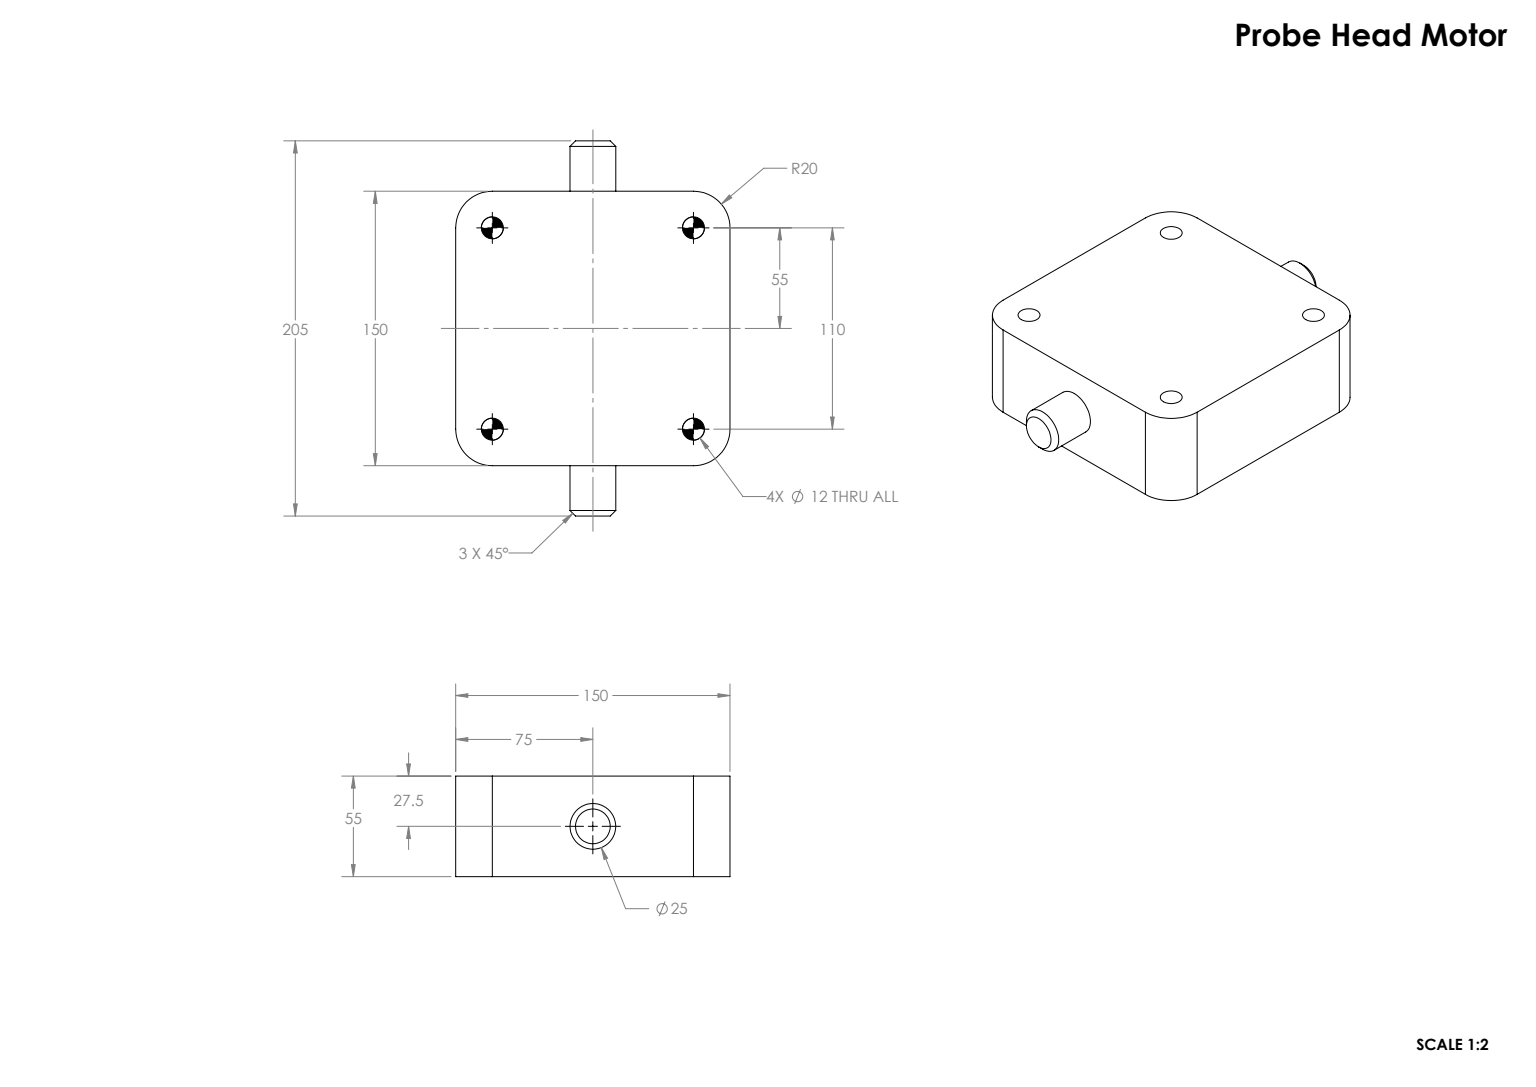
ISO-10303-21;
HEADER;
FILE_DESCRIPTION (('STEP AP214'),
    '1' );
FILE_NAME ('Probe head motor.step',
    '2026-10-28T15:55:38',
    ( '' ),
    ( '' ),
    'SwSTEP 2.0',
    'SolidWorks 2025',
    '' );
FILE_SCHEMA (( 'AUTOMOTIVE_DESIGN' ));
ENDSEC;

DATA;
#16=EDGE_LOOP ( 'NONE', ( #280, #1989 ) ) ;
#35=DIRECTION ( 'NONE',  ( 1.000000000000000000, 0.000000000000000000, 0.000000000000000000 ) ) ;
#37=DIRECTION ( 'NONE',  ( -0.000000000000000000, -0.000000000000000000, 1.000000000000000000 ) ) ;
#50=VECTOR ( 'NONE', #966, 1000.000000000000000 ) ;
#53=CARTESIAN_POINT ( 'NONE',  ( 54.99999999999999289, -55.00000000000000711, 27.50000000000000000 ) ) ;
#58=DIRECTION ( 'NONE',  ( 1.000000000000000000, 0.000000000000000000, 0.000000000000000000 ) ) ;
#59=ORIENTED_EDGE ( 'NONE', *, *, #4247, .T. ) ;
#60=CARTESIAN_POINT ( 'NONE',  ( -75.00000000000000000, 0.000000000000000000, 0.000000000000000000 ) ) ;
#66=VERTEX_POINT ( 'NONE', #5954 ) ;
#75=DIRECTION ( 'NONE',  ( -0.000000000000000000, -0.000000000000000000, -1.000000000000000000 ) ) ;
#86=CIRCLE ( 'NONE', #779, 5.999999999999984901 ) ;
#101=ORIENTED_EDGE ( 'NONE', *, *, #2517, .F. ) ;
#110=VERTEX_POINT ( 'NONE', #3400 ) ;
#138=EDGE_LOOP ( 'NONE', ( #2116, #5136, #6924, #3116 ) ) ;
#142=ORIENTED_EDGE ( 'NONE', *, *, #1025, .T. ) ;
#158=PLANE ( 'NONE',  #296 ) ;
#191=ORIENTED_EDGE ( 'NONE', *, *, #863, .F. ) ;
#192=DIRECTION ( 'NONE',  ( 1.000000000000000000, 0.000000000000000000, 0.000000000000000000 ) ) ;
#200=CARTESIAN_POINT ( 'NONE',  ( 75.00000000000000000, 55.00000000000000711, 27.50000000000000000 ) ) ;
#209=AXIS2_PLACEMENT_3D ( 'NONE', #1275, #5067, #1401 ) ;
#220=DIRECTION ( 'NONE',  ( 1.000000000000000000, 0.000000000000000000, 0.000000000000000000 ) ) ;
#236=CIRCLE ( 'NONE', #5782, 12.50000000000000000 ) ;
#241=EDGE_CURVE ( 'NONE', #7110, #7555, #6784, .T. ) ;
#246=FACE_OUTER_BOUND ( 'NONE', #495, .T. ) ;
#257=LINE ( 'NONE', #1580, #7553 ) ;
#275=ORIENTED_EDGE ( 'NONE', *, *, #5871, .F. ) ;
#277=AXIS2_PLACEMENT_3D ( 'NONE', #5185, #677, #1430 ) ;
#280=ORIENTED_EDGE ( 'NONE', *, *, #241, .T. ) ;
#288=DIRECTION ( 'NONE',  ( 0.000000000000000000, 0.000000000000000000, 1.000000000000000000 ) ) ;
#296=AXIS2_PLACEMENT_3D ( 'NONE', #5951, #1969, #3246 ) ;
#301=ORIENTED_EDGE ( 'NONE', *, *, #715, .F. ) ;
#316=CARTESIAN_POINT ( 'NONE',  ( 54.99999999999999289, 55.00000000000000711, 27.50000000000000000 ) ) ;
#339=CARTESIAN_POINT ( 'NONE',  ( -75.00000000000000000, -75.00000000000000000, -27.50000000000000000 ) ) ;
#340=ORIENTED_EDGE ( 'NONE', *, *, #1134, .T. ) ;
#356=AXIS2_PLACEMENT_3D ( 'NONE', #3494, #2749, #5417 ) ;
#382=CARTESIAN_POINT ( 'NONE',  ( -54.99999999999999289, 55.00000000000000711, 27.50000000000000000 ) ) ;
#384=CIRCLE ( 'NONE', #1751, 5.999999999999984901 ) ;
#388=ORIENTED_EDGE ( 'NONE', *, *, #3277, .T. ) ;
#395=DIRECTION ( 'NONE',  ( -0.000000000000000000, -0.000000000000000000, 1.000000000000000000 ) ) ;
#420=CARTESIAN_POINT ( 'NONE',  ( -102.5000000000000000, 0.000000000000000000, -9.500000000000008882 ) ) ;
#437=DIRECTION ( 'NONE',  ( 0.000000000000000000, 0.000000000000000000, -1.000000000000000000 ) ) ;
#453=CARTESIAN_POINT ( 'NONE',  ( -75.00000000000000000, 55.00000000000000711, 27.50000000000000000 ) ) ;
#494=CARTESIAN_POINT ( 'NONE',  ( -75.00000000000000000, 1.530808498934191521E-15, -12.50000000000000000 ) ) ;
#495=EDGE_LOOP ( 'NONE', ( #2773, #191, #1926, #6706 ) ) ;
#499=ORIENTED_EDGE ( 'NONE', *, *, #1382, .F. ) ;
#512=EDGE_CURVE ( 'NONE', #554, #2252, #3311, .T. ) ;
#518=FACE_OUTER_BOUND ( 'NONE', #6089, .T. ) ;
#527=CARTESIAN_POINT ( 'NONE',  ( 54.99999999999999289, -55.00000000000000711, -27.50000000000000000 ) ) ;
#531=DIRECTION ( 'NONE',  ( 1.000000000000000000, 0.000000000000000000, 0.000000000000000000 ) ) ;
#532=DIRECTION ( 'NONE',  ( 0.000000000000000000, 0.000000000000000000, -1.000000000000000000 ) ) ;
#550=SHAPE_DEFINITION_REPRESENTATION ( #6549, #5477 ) ;
#554=VERTEX_POINT ( 'NONE', #494 ) ;
#582=DIRECTION ( 'NONE',  ( 0.7071067811865487940, 0.000000000000000000, -0.7071067811865463515 ) ) ;
#585=ORIENTED_EDGE ( 'NONE', *, *, #8135, .F. ) ;
#596=ORIENTED_EDGE ( 'NONE', *, *, #2034, .T. ) ;
#598=AXIS2_PLACEMENT_3D ( 'NONE', #1970, #37, #7220 ) ;
#614=DIRECTION ( 'NONE',  ( 1.000000000000000000, 0.000000000000000000, 0.000000000000000000 ) ) ;
#617=ADVANCED_FACE ( 'NONE', ( #5555 ), #6947, .T. ) ;
#641=ORIENTED_EDGE ( 'NONE', *, *, #6036, .F. ) ;
#652=AXIS2_PLACEMENT_3D ( 'NONE', #316, #3056, #8044 ) ;
#674=FACE_OUTER_BOUND ( 'NONE', #5673, .T. ) ;
#677=DIRECTION ( 'NONE',  ( 1.000000000000000000, 0.000000000000000000, 0.000000000000000000 ) ) ;
#693=FACE_OUTER_BOUND ( 'NONE', #2495, .T. ) ;
#715=EDGE_CURVE ( 'NONE', #3072, #2500, #2204, .T. ) ;
#723=ORIENTED_EDGE ( 'NONE', *, *, #8302, .T. ) ;
#734=EDGE_LOOP ( 'NONE', ( #5853, #4869 ) ) ;
#752=CARTESIAN_POINT ( 'NONE',  ( -54.99999999999999289, 75.00000000000000000, 27.50000000000000000 ) ) ;
#760=ORIENTED_EDGE ( 'NONE', *, *, #7716, .F. ) ;
#764=EDGE_LOOP ( 'NONE', ( #7104, #4270, #4312, #1914 ) ) ;
#773=CYLINDRICAL_SURFACE ( 'NONE', #4839, 5.999999999999991118 ) ;
#779=AXIS2_PLACEMENT_3D ( 'NONE', #7723, #2681, #5258 ) ;
#796=ORIENTED_EDGE ( 'NONE', *, *, #4247, .F. ) ;
#807=CONICAL_SURFACE ( 'NONE', #951, 12.50000000000000000, 0.7853981633974560506 ) ;
#808=AXIS2_PLACEMENT_3D ( 'NONE', #888, #4718, #2129 ) ;
#812=ORIENTED_EDGE ( 'NONE', *, *, #1185, .F. ) ;
#828=CARTESIAN_POINT ( 'NONE',  ( 75.00000000000000000, 55.00000000000000711, -27.50000000000000000 ) ) ;
#836=VERTEX_POINT ( 'NONE', #6820 ) ;
#847=DIRECTION ( 'NONE',  ( 0.000000000000000000, 0.000000000000000000, 1.000000000000000000 ) ) ;
#848=CIRCLE ( 'NONE', #1394, 5.999999999999991118 ) ;
#863=EDGE_CURVE ( 'NONE', #7276, #4717, #4483, .T. ) ;
#885=EDGE_CURVE ( 'NONE', #1626, #6639, #3839, .T. ) ;
#888=CARTESIAN_POINT ( 'NONE',  ( -54.99999999999999289, -55.00000000000000711, 27.50000000000000000 ) ) ;
#912=CARTESIAN_POINT ( 'NONE',  ( -54.99999999999999289, 55.00000000000000711, -27.50000000000000000 ) ) ;
#914=ORIENTED_EDGE ( 'NONE', *, *, #3174, .T. ) ;
#921=EDGE_CURVE ( 'NONE', #3696, #7524, #4657, .T. ) ;
#928=CIRCLE ( 'NONE', #1205, 5.999999999999991118 ) ;
#951=AXIS2_PLACEMENT_3D ( 'NONE', #3629, #2188, #7493 ) ;
#956=EDGE_LOOP ( 'NONE', ( #1669, #2525 ) ) ;
#965=DIRECTION ( 'NONE',  ( -1.000000000000000000, 0.000000000000000000, 0.000000000000000000 ) ) ;
#966=DIRECTION ( 'NONE',  ( -0.000000000000000000, -0.000000000000000000, 1.000000000000000000 ) ) ;
#976=ORIENTED_EDGE ( 'NONE', *, *, #1235, .T. ) ;
#988=DIRECTION ( 'NONE',  ( -0.000000000000000000, -0.000000000000000000, 1.000000000000000000 ) ) ;
#1025=EDGE_CURVE ( 'NONE', #6358, #4954, #6815, .T. ) ;
#1060=AXIS2_PLACEMENT_3D ( 'NONE', #3558, #6825, #1679 ) ;
#1064=ORIENTED_EDGE ( 'NONE', *, *, #1543, .F. ) ;
#1066=AXIS2_PLACEMENT_3D ( 'NONE', #60, #2652, #5223 ) ;
#1068=CARTESIAN_POINT ( 'NONE',  ( -60.99999999999998579, -55.00000000000000711, 27.50000000000000000 ) ) ;
#1073=AXIS2_PLACEMENT_3D ( 'NONE', #4907, #6004, #220 ) ;
#1075=ADVANCED_FACE ( 'NONE', ( #7748 ), #1882, .T. ) ;
#1117=LINE ( 'NONE', #2431, #6840 ) ;
#1134=EDGE_CURVE ( 'NONE', #5699, #3094, #5750, .T. ) ;
#1149=DIRECTION ( 'NONE',  ( -1.000000000000000000, 0.000000000000000000, 0.000000000000000000 ) ) ;
#1152=CARTESIAN_POINT ( 'NONE',  ( 60.99999999999998579, -55.00000000000000711, 27.50000000000000000 ) ) ;
#1159=PLANE ( 'NONE',  #4129 ) ;
#1169=CARTESIAN_POINT ( 'NONE',  ( 102.5000000000000000, 0.000000000000000000, 12.50000000000000000 ) ) ;
#1177=CIRCLE ( 'NONE', #2781, 5.999999999999984901 ) ;
#1185=EDGE_CURVE ( 'NONE', #8175, #4245, #7456, .T. ) ;
#1205=AXIS2_PLACEMENT_3D ( 'NONE', #2733, #7214, #192 ) ;
#1214=AXIS2_PLACEMENT_3D ( 'NONE', #912, #6734, #4258 ) ;
#1216=DIRECTION ( 'NONE',  ( -1.000000000000000000, 0.000000000000000000, 0.000000000000000000 ) ) ;
#1222=VECTOR ( 'NONE', #4044, 1000.000000000000000 ) ;
#1235=EDGE_CURVE ( 'NONE', #6452, #7276, #5560, .T. ) ;
#1275=CARTESIAN_POINT ( 'NONE',  ( -102.5000000000000000, 0.000000000000000000, 0.000000000000000000 ) ) ;
#1292=DIRECTION ( 'NONE',  ( -0.000000000000000000, -0.000000000000000000, 1.000000000000000000 ) ) ;
#1295=EDGE_LOOP ( 'NONE', ( #5051, #4898, #3815, #4605 ) ) ;
#1299=AXIS2_PLACEMENT_3D ( 'NONE', #5884, #1507, #5927 ) ;
#1309=STYLED_ITEM('',(#8386),#3442);
#1316=ORIENTED_EDGE ( 'NONE', *, *, #5149, .T. ) ;
#1341=EDGE_LOOP ( 'NONE', ( #3743, #2060, #2905, #3577 ) ) ;
#1361=CARTESIAN_POINT ( 'NONE',  ( -102.5000000000000000, 1.347111479062088996E-15, 9.500000000000008882 ) ) ;
#1363=ORIENTED_EDGE ( 'NONE', *, *, #7635, .T. ) ;
#1377=DIRECTION ( 'NONE',  ( 0.000000000000000000, 0.000000000000000000, -1.000000000000000000 ) ) ;
#1378=CYLINDRICAL_SURFACE ( 'NONE', #2162, 5.999999999999991118 ) ;
#1382=EDGE_CURVE ( 'NONE', #7568, #7256, #5423, .T. ) ;
#1386=EDGE_LOOP ( 'NONE', ( #5814, #142 ) ) ;
#1392=EDGE_CURVE ( 'NONE', #4954, #2252, #6357, .T. ) ;
#1394=AXIS2_PLACEMENT_3D ( 'NONE', #2395, #3731, #6308 ) ;
#1398=ORIENTED_EDGE ( 'NONE', *, *, #1382, .T. ) ;
#1399=DIRECTION ( 'NONE',  ( -0.000000000000000000, -0.000000000000000000, 1.000000000000000000 ) ) ;
#1401=DIRECTION ( 'NONE',  ( 0.000000000000000000, 0.000000000000000000, 1.000000000000000000 ) ) ;
#1405=DIRECTION ( 'NONE',  ( 0.7071067811865487940, 8.659560562354918067E-17, 0.7071067811865463515 ) ) ;
#1406=FACE_OUTER_BOUND ( 'NONE', #6060, .T. ) ;
#1407=CARTESIAN_POINT ( 'NONE',  ( -75.00000000000000000, 55.00000000000000711, -27.50000000000000000 ) ) ;
#1430=DIRECTION ( 'NONE',  ( 0.000000000000000000, 0.000000000000000000, 1.000000000000000000 ) ) ;
#1433=VECTOR ( 'NONE', #5737, 1000.000000000000000 ) ;
#1434=FACE_OUTER_BOUND ( 'NONE', #2226, .T. ) ;
#1449=DIRECTION ( 'NONE',  ( 1.000000000000000000, 0.000000000000000000, -0.000000000000000000 ) ) ;
#1460=AXIS2_PLACEMENT_3D ( 'NONE', #7776, #8199, #6245 ) ;
#1461=DIRECTION ( 'NONE',  ( 1.000000000000000000, 0.000000000000000000, 0.000000000000000000 ) ) ;
#1472=VECTOR ( 'NONE', #4316, 1000.000000000000000 ) ;
#1476=EDGE_LOOP ( 'NONE', ( #4624, #1316 ) ) ;
#1482=PLANE ( 'NONE',  #4550 ) ;
#1492=DIRECTION ( 'NONE',  ( 1.000000000000000000, 0.000000000000000000, 0.000000000000000000 ) ) ;
#1498=ADVANCED_FACE ( 'NONE', ( #4662 ), #3983, .F. ) ;
#1507=DIRECTION ( 'NONE',  ( 0.000000000000000000, 0.000000000000000000, 1.000000000000000000 ) ) ;
#1523=LINE ( 'NONE', #4077, #6033 ) ;
#1542=EDGE_CURVE ( 'NONE', #7555, #4076, #4780, .T. ) ;
#1543=EDGE_CURVE ( 'NONE', #3044, #6339, #848, .T. ) ;
#1565=CARTESIAN_POINT ( 'NONE',  ( 102.5000000000000000, 0.000000000000000000, 12.50000000000000000 ) ) ;
#1572=AXIS2_PLACEMENT_3D ( 'NONE', #3282, #1924, #5869 ) ;
#1580=CARTESIAN_POINT ( 'NONE',  ( 99.49999999999998579, 1.530808498934191521E-15, -12.50000000000000000 ) ) ;
#1585=PRODUCT_DEFINITION ( 'UNKNOWN', '', #8277, #4878 ) ;
#1586=AXIS2_PLACEMENT_3D ( 'NONE', #2848, #5393, #6777 ) ;
#1589=DIRECTION ( 'NONE',  ( 1.000000000000000000, 0.000000000000000000, 0.000000000000000000 ) ) ;
#1599=AXIS2_PLACEMENT_3D ( 'NONE', #7278, #2142, #6512 ) ;
#1609=ORIENTED_EDGE ( 'NONE', *, *, #6476, .F. ) ;
#1619=ORIENTED_EDGE ( 'NONE', *, *, #2976, .F. ) ;
#1625=DIRECTION ( 'NONE',  ( 1.000000000000000000, 0.000000000000000000, 0.000000000000000000 ) ) ;
#1626=VERTEX_POINT ( 'NONE', #5552 ) ;
#1635=DIRECTION ( 'NONE',  ( -0.000000000000000000, -0.000000000000000000, -1.000000000000000000 ) ) ;
#1654=ORIENTED_EDGE ( 'NONE', *, *, #2229, .F. ) ;
#1657=ORIENTED_EDGE ( 'NONE', *, *, #1392, .T. ) ;
#1661=LINE ( 'NONE', #339, #5798 ) ;
#1663=ADVANCED_FACE ( 'NONE', ( #3888, #2011, #6544, #5286, #3359 ), #158, .F. ) ;
#1669=ORIENTED_EDGE ( 'NONE', *, *, #6182, .F. ) ;
#1675=CARTESIAN_POINT ( 'NONE',  ( -75.00000000000000000, -54.99999999999999289, 27.50000000000000000 ) ) ;
#1679=DIRECTION ( 'NONE',  ( 0.000000000000000000, 0.000000000000000000, -1.000000000000000000 ) ) ;
#1685=DIRECTION ( 'NONE',  ( -0.000000000000000000, -1.000000000000000000, -0.000000000000000000 ) ) ;
#1689=ORIENTED_EDGE ( 'NONE', *, *, #6534, .T. ) ;
#1694=DIRECTION ( 'NONE',  ( 1.000000000000000000, 0.000000000000000000, 0.000000000000000000 ) ) ;
#1696=ORIENTED_EDGE ( 'NONE', *, *, #715, .T. ) ;
#1715=CIRCLE ( 'NONE', #7657, 5.999999999999991118 ) ;
#1724=ORIENTED_EDGE ( 'NONE', *, *, #5346, .T. ) ;
#1731=EDGE_LOOP ( 'NONE', ( #7387, #5133, #8189, #1619 ) ) ;
#1749=DIRECTION ( 'NONE',  ( 1.000000000000000000, 0.000000000000000000, 0.000000000000000000 ) ) ;
#1751=AXIS2_PLACEMENT_3D ( 'NONE', #1805, #2063, #7837 ) ;
#1765=LINE ( 'NONE', #6220, #6456 ) ;
#1774=CARTESIAN_POINT ( 'NONE',  ( 102.5000000000000000, 0.000000000000000000, 12.50000000000000000 ) ) ;
#1777=FACE_OUTER_BOUND ( 'NONE', #3624, .T. ) ;
#1800=VECTOR ( 'NONE', #4904, 1000.000000000000000 ) ;
#1805=CARTESIAN_POINT ( 'NONE',  ( 54.99999999999999289, 55.00000000000000711, -27.50000000000000000 ) ) ;
#1829=ADVANCED_FACE ( 'NONE', ( #5289, #5255 ), #3937, .F. ) ;
#1867=EDGE_CURVE ( 'NONE', #8175, #3044, #4291, .T. ) ;
#1882=PLANE ( 'NONE',  #1572 ) ;
#1913=VECTOR ( 'NONE', #8057, 1000.000000000000000 ) ;
#1914=ORIENTED_EDGE ( 'NONE', *, *, #5462, .F. ) ;
#1924=DIRECTION ( 'NONE',  ( -1.000000000000000000, 0.000000000000000000, -0.000000000000000000 ) ) ;
#1926=ORIENTED_EDGE ( 'NONE', *, *, #1235, .F. ) ;
#1927=VECTOR ( 'NONE', #2123, 1000.000000000000000 ) ;
#1930=ADVANCED_FACE ( 'NONE', ( #7832 ), #6986, .T. ) ;
#1948=ORIENTED_EDGE ( 'NONE', *, *, #885, .F. ) ;
#1959=ORIENTED_EDGE ( 'NONE', *, *, #2080, .T. ) ;
#1969=DIRECTION ( 'NONE',  ( 0.000000000000000000, 0.000000000000000000, 1.000000000000000000 ) ) ;
#1970=CARTESIAN_POINT ( 'NONE',  ( 54.99999999999999289, -55.00000000000000711, -27.50000000000000000 ) ) ;
#1973=CARTESIAN_POINT ( 'NONE',  ( -49.00000000000000000, 55.00000000000000711, 27.50000000000000000 ) ) ;
#1976=EDGE_CURVE ( 'NONE', #66, #5533, #7130, .T. ) ;
#1980=EDGE_CURVE ( 'NONE', #7524, #2265, #2627, .T. ) ;
#1983=DIRECTION ( 'NONE',  ( 0.000000000000000000, 0.000000000000000000, 1.000000000000000000 ) ) ;
#1985=CARTESIAN_POINT ( 'NONE',  ( -54.99999999999999289, 55.00000000000000711, -27.50000000000000000 ) ) ;
#1989=ORIENTED_EDGE ( 'NONE', *, *, #4023, .T. ) ;
#1996=CIRCLE ( 'NONE', #3715, 12.50000000000000000 ) ;
#2000=CARTESIAN_POINT ( 'NONE',  ( -54.99999999999999289, 55.00000000000000711, -27.50000000000000000 ) ) ;
#2011=FACE_BOUND ( 'NONE', #2386, .T. ) ;
#2018=ADVANCED_FACE ( 'NONE', ( #4678, #7262 ), #1482, .F. ) ;
#2028=AXIS2_PLACEMENT_3D ( 'NONE', #8099, #3603, #7469 ) ;
#2034=EDGE_CURVE ( 'NONE', #6639, #2500, #5444, .T. ) ;
#2047=CARTESIAN_POINT ( 'NONE',  ( -60.99999999999998579, -55.00000000000000711, 27.50000000000000000 ) ) ;
#2053=DIRECTION ( 'NONE',  ( -1.000000000000000000, -0.000000000000000000, -0.000000000000000000 ) ) ;
#2060=ORIENTED_EDGE ( 'NONE', *, *, #6540, .T. ) ;
#2063=DIRECTION ( 'NONE',  ( -0.000000000000000000, -0.000000000000000000, 1.000000000000000000 ) ) ;
#2066=ORIENTED_EDGE ( 'NONE', *, *, #7515, .F. ) ;
#2076=CARTESIAN_POINT ( 'NONE',  ( 75.00000000000000000, 0.000000000000000000, 0.000000000000000000 ) ) ;
#2080=EDGE_CURVE ( 'NONE', #3696, #2372, #2373, .T. ) ;
#2110=CARTESIAN_POINT ( 'NONE',  ( -60.99999999999997868, 55.00000000000000711, -27.50000000000000000 ) ) ;
#2116=ORIENTED_EDGE ( 'NONE', *, *, #4902, .F. ) ;
#2123=DIRECTION ( 'NONE',  ( 0.000000000000000000, 1.000000000000000000, 0.000000000000000000 ) ) ;
#2126=DIRECTION ( 'NONE',  ( -1.000000000000000000, -0.000000000000000000, -0.000000000000000000 ) ) ;
#2129=DIRECTION ( 'NONE',  ( 1.000000000000000000, 0.000000000000000000, 0.000000000000000000 ) ) ;
#2134=AXIS2_PLACEMENT_3D ( 'NONE', #8300, #6470, #614 ) ;
#2138=DIRECTION ( 'NONE',  ( 1.000000000000000000, 0.000000000000000000, 0.000000000000000000 ) ) ;
#2142=DIRECTION ( 'NONE',  ( 1.000000000000000000, 0.000000000000000000, 0.000000000000000000 ) ) ;
#2146=( NAMED_UNIT ( * ) SI_UNIT ( $, .STERADIAN. ) SOLID_ANGLE_UNIT ( ) );
#2150=ORIENTED_EDGE ( 'NONE', *, *, #1542, .F. ) ;
#2162=AXIS2_PLACEMENT_3D ( 'NONE', #53, #5882, #7285 ) ;
#2166=DIRECTION ( 'NONE',  ( 0.000000000000000000, 0.000000000000000000, 1.000000000000000000 ) ) ;
#2188=DIRECTION ( 'NONE',  ( -1.000000000000000000, -0.000000000000000000, -0.000000000000000000 ) ) ;
#2195=DIRECTION ( 'NONE',  ( -0.000000000000000000, -0.000000000000000000, 1.000000000000000000 ) ) ;
#2202=DIRECTION ( 'NONE',  ( -0.000000000000000000, -1.000000000000000000, -0.000000000000000000 ) ) ;
#2204=LINE ( 'NONE', #1675, #50 ) ;
#2223=FACE_BOUND ( 'NONE', #7249, .T. ) ;
#2226=EDGE_LOOP ( 'NONE', ( #2246, #7149, #4337, #6802 ) ) ;
#2229=EDGE_CURVE ( 'NONE', #5699, #7276, #6330, .T. ) ;
#2235=ORIENTED_EDGE ( 'NONE', *, *, #1867, .T. ) ;
#2246=ORIENTED_EDGE ( 'NONE', *, *, #6540, .F. ) ;
#2252=VERTEX_POINT ( 'NONE', #4669 ) ;
#2265=VERTEX_POINT ( 'NONE', #7253 ) ;
#2267=DIRECTION ( 'NONE',  ( 0.000000000000000000, 1.000000000000000000, 0.000000000000000000 ) ) ;
#2269=CARTESIAN_POINT ( 'NONE',  ( -54.99999999999999289, -54.99999999999999289, 27.50000000000000000 ) ) ;
#2270=EDGE_LOOP ( 'NONE', ( #5470, #1064 ) ) ;
#2315=CYLINDRICAL_SURFACE ( 'NONE', #1073, 5.999999999999991118 ) ;
#2337=AXIS2_PLACEMENT_3D ( 'NONE', #3997, #5908, #4801 ) ;
#2345=EDGE_CURVE ( 'NONE', #2252, #7231, #4050, .T. ) ;
#2346=EDGE_LOOP ( 'NONE', ( #8111, #6761 ) ) ;
#2348=EDGE_CURVE ( 'NONE', #6145, #8000, #1996, .T. ) ;
#2372=VERTEX_POINT ( 'NONE', #5312 ) ;
#2373=LINE ( 'NONE', #3563, #1913 ) ;
#2384=ORIENTED_EDGE ( 'NONE', *, *, #4773, .F. ) ;
#2386=EDGE_LOOP ( 'NONE', ( #59, #3390 ) ) ;
#2395=CARTESIAN_POINT ( 'NONE',  ( -54.99999999999999289, -55.00000000000000711, 27.50000000000000000 ) ) ;
#2431=CARTESIAN_POINT ( 'NONE',  ( -75.00000000000000000, 75.00000000000000000, 27.50000000000000000 ) ) ;
#2435=ORIENTED_EDGE ( 'NONE', *, *, #8135, .T. ) ;
#2456=DIRECTION ( 'NONE',  ( -0.7071067811865420216, 0.000000000000000000, 0.7071067811865531239 ) ) ;
#2463=ORIENTED_EDGE ( 'NONE', *, *, #1980, .T. ) ;
#2465=ORIENTED_EDGE ( 'NONE', *, *, #3174, .F. ) ;
#2466=CARTESIAN_POINT ( 'NONE',  ( -49.00000000000000000, -55.00000000000000711, 27.50000000000000000 ) ) ;
#2480=CARTESIAN_POINT ( 'NONE',  ( -75.00000000000000000, 0.000000000000000000, 12.50000000000000000 ) ) ;
#2488=DIRECTION ( 'NONE',  ( -0.000000000000000000, -0.000000000000000000, 1.000000000000000000 ) ) ;
#2495=EDGE_LOOP ( 'NONE', ( #4227, #7457, #7004, #2728 ) ) ;
#2500=VERTEX_POINT ( 'NONE', #7466 ) ;
#2517=EDGE_CURVE ( 'NONE', #4954, #6358, #2712, .T. ) ;
#2525=ORIENTED_EDGE ( 'NONE', *, *, #3782, .F. ) ;
#2526=CARTESIAN_POINT ( 'NONE',  ( -102.5000000000000000, 0.000000000000000000, -9.500000000000008882 ) ) ;
#2538=CIRCLE ( 'NONE', #7244, 5.999999999999991118 ) ;
#2558=ORIENTED_EDGE ( 'NONE', *, *, #3873, .F. ) ;
#2595=LINE ( 'NONE', #1973, #6878 ) ;
#2627=LINE ( 'NONE', #3996, #2932 ) ;
#2635=DIRECTION ( 'NONE',  ( -0.000000000000000000, -0.000000000000000000, 1.000000000000000000 ) ) ;
#2652=DIRECTION ( 'NONE',  ( 1.000000000000000000, 0.000000000000000000, 0.000000000000000000 ) ) ;
#2656=CARTESIAN_POINT ( 'NONE',  ( 55.00000000000000711, -75.00000000000000000, -27.50000000000000000 ) ) ;
#2664=DIRECTION ( 'NONE',  ( 0.000000000000000000, 0.000000000000000000, 1.000000000000000000 ) ) ;
#2673=CARTESIAN_POINT ( 'NONE',  ( 102.5000000000000000, 0.000000000000000000, 0.000000000000000000 ) ) ;
#2677=AXIS2_PLACEMENT_3D ( 'NONE', #4426, #7098, #5199 ) ;
#2681=DIRECTION ( 'NONE',  ( -0.000000000000000000, -0.000000000000000000, 1.000000000000000000 ) ) ;
#2686=AXIS2_PLACEMENT_3D ( 'NONE', #3148, #3792, #6322 ) ;
#2699=CIRCLE ( 'NONE', #808, 5.999999999999991118 ) ;
#2712=CIRCLE ( 'NONE', #1586, 9.500000000000008882 ) ;
#2722=CARTESIAN_POINT ( 'NONE',  ( 49.00000000000000000, -55.00000000000000711, 27.50000000000000000 ) ) ;
#2728=ORIENTED_EDGE ( 'NONE', *, *, #3761, .F. ) ;
#2731=LINE ( 'NONE', #752, #7531 ) ;
#2733=CARTESIAN_POINT ( 'NONE',  ( 54.99999999999999289, -55.00000000000000711, 27.50000000000000000 ) ) ;
#2737=CARTESIAN_POINT ( 'NONE',  ( 54.99999999999999289, -54.99999999999999289, 27.50000000000000000 ) ) ;
#2749=DIRECTION ( 'NONE',  ( 0.000000000000000000, 0.000000000000000000, 1.000000000000000000 ) ) ;
#2773=ORIENTED_EDGE ( 'NONE', *, *, #4299, .F. ) ;
#2781=AXIS2_PLACEMENT_3D ( 'NONE', #527, #395, #4256 ) ;
#2799=CONICAL_SURFACE ( 'NONE', #8058, 12.50000000000000000, 0.7853981633974560506 ) ;
#2801=AXIS2_PLACEMENT_3D ( 'NONE', #5240, #3928, #6497 ) ;
#2808=VECTOR ( 'NONE', #2456, 999.9999999999998863 ) ;
#2817=LINE ( 'NONE', #1565, #4522 ) ;
#2818=CIRCLE ( 'NONE', #7413, 5.999999999999991118 ) ;
#2819=AXIS2_PLACEMENT_3D ( 'NONE', #6539, #3393, #3314 ) ;
#2824=AXIS2_PLACEMENT_3D ( 'NONE', #2000, #8279, #4534 ) ;
#2827=DIRECTION ( 'NONE',  ( -0.000000000000000000, -0.000000000000000000, 1.000000000000000000 ) ) ;
#2829=CARTESIAN_POINT ( 'NONE',  ( -60.99999999999998579, 55.00000000000000711, 27.50000000000000000 ) ) ;
#2848=CARTESIAN_POINT ( 'NONE',  ( -102.5000000000000000, 0.000000000000000000, 0.000000000000000000 ) ) ;
#2856=EDGE_LOOP ( 'NONE', ( #7495, #6405, #5755, #3429 ) ) ;
#2863=DIRECTION ( 'NONE',  ( 1.000000000000000000, 0.000000000000000000, 0.000000000000000000 ) ) ;
#2878=AXIS2_PLACEMENT_3D ( 'NONE', #6082, #4777, #6611 ) ;
#2883=CARTESIAN_POINT ( 'NONE',  ( -54.99999999999999289, -54.99999999999999289, -27.50000000000000000 ) ) ;
#2894=CARTESIAN_POINT ( 'NONE',  ( 54.99999999999999289, 55.00000000000000711, 27.50000000000000000 ) ) ;
#2905=ORIENTED_EDGE ( 'NONE', *, *, #2348, .F. ) ;
#2911=DIRECTION ( 'NONE',  ( 1.000000000000000000, 0.000000000000000000, 0.000000000000000000 ) ) ;
#2932=VECTOR ( 'NONE', #1399, 1000.000000000000000 ) ;
#2941=ORIENTED_EDGE ( 'NONE', *, *, #5514, .F. ) ;
#2976=EDGE_CURVE ( 'NONE', #7110, #8191, #5228, .T. ) ;
#2985=ORIENTED_EDGE ( 'NONE', *, *, #241, .F. ) ;
#2992=CARTESIAN_POINT ( 'NONE',  ( 55.00000000000000711, 75.00000000000000000, 27.50000000000000000 ) ) ;
#3044=VERTEX_POINT ( 'NONE', #2047 ) ;
#3055=CYLINDRICAL_SURFACE ( 'NONE', #6596, 20.00000000000000355 ) ;
#3056=DIRECTION ( 'NONE',  ( -0.000000000000000000, -0.000000000000000000, 1.000000000000000000 ) ) ;
#3072=VERTEX_POINT ( 'NONE', #3670 ) ;
#3074=ADVANCED_FACE ( 'NONE', ( #674 ), #7169, .F. ) ;
#3088=ORIENTED_EDGE ( 'NONE', *, *, #1025, .F. ) ;
#3094=VERTEX_POINT ( 'NONE', #2656 ) ;
#3100=ORIENTED_EDGE ( 'NONE', *, *, #6902, .F. ) ;
#3101=VECTOR ( 'NONE', #1685, 1000.000000000000000 ) ;
#3105=DIRECTION ( 'NONE',  ( 0.000000000000000000, 0.000000000000000000, -1.000000000000000000 ) ) ;
#3116=ORIENTED_EDGE ( 'NONE', *, *, #4151, .T. ) ;
#3139=CARTESIAN_POINT ( 'NONE',  ( 102.5000000000000000, 1.347111479062085446E-15, -9.499999999999952038 ) ) ;
#3148=CARTESIAN_POINT ( 'NONE',  ( -99.49999999999998579, 0.000000000000000000, 0.000000000000000000 ) ) ;
#3151=LINE ( 'NONE', #3748, #1433 ) ;
#3171=CIRCLE ( 'NONE', #7910, 5.999999999999984901 ) ;
#3173=CONICAL_SURFACE ( 'NONE', #7653, 9.500000000000008882, 0.7853981633974466137 ) ;
#3174=EDGE_CURVE ( 'NONE', #7809, #1626, #2731, .T. ) ;
#3186=EDGE_LOOP ( 'NONE', ( #3088, #6469, #3532, #4873 ) ) ;
#3221=VECTOR ( 'NONE', #5579, 1000.000000000000000 ) ;
#3246=DIRECTION ( 'NONE',  ( 1.000000000000000000, 0.000000000000000000, -0.000000000000000000 ) ) ;
#3249=CYLINDRICAL_SURFACE ( 'NONE', #3777, 12.50000000000000000 ) ;
#3262=ORIENTED_EDGE ( 'NONE', *, *, #4902, .T. ) ;
#3277=EDGE_CURVE ( 'NONE', #7206, #3072, #6028, .T. ) ;
#3280=CARTESIAN_POINT ( 'NONE',  ( -49.00000000000000711, 55.00000000000000711, -27.50000000000000000 ) ) ;
#3282=CARTESIAN_POINT ( 'NONE',  ( -102.5000000000000000, 0.000000000000000000, 12.50000000000000000 ) ) ;
#3286=ADVANCED_FACE ( 'NONE', ( #5558 ), #7591, .F. ) ;
#3295=ADVANCED_FACE ( 'NONE', ( #3553 ), #4311, .T. ) ;
#3311=LINE ( 'NONE', #3700, #3405 ) ;
#3314=DIRECTION ( 'NONE',  ( 0.000000000000000000, 0.000000000000000000, -1.000000000000000000 ) ) ;
#3322=CARTESIAN_POINT ( 'NONE',  ( -102.5000000000000000, 1.163414459189986668E-15, 9.500000000000008882 ) ) ;
#3324=AXIS2_PLACEMENT_3D ( 'NONE', #7462, #5642, #965 ) ;
#3325=CARTESIAN_POINT ( 'NONE',  ( 0.000000000000000000, 0.000000000000000000, 27.50000000000000000 ) ) ;
#3348=CIRCLE ( 'NONE', #3904, 20.00000000000000355 ) ;
#3359=FACE_OUTER_BOUND ( 'NONE', #5904, .T. ) ;
#3368=ORIENTED_EDGE ( 'NONE', *, *, #7209, .F. ) ;
#3371=FACE_OUTER_BOUND ( 'NONE', #2856, .T. ) ;
#3378=ADVANCED_FACE ( 'NONE', ( #3822 ), #3173, .T. ) ;
#3379=( NAMED_UNIT ( * ) SI_UNIT ( $, .STERADIAN. ) SOLID_ANGLE_UNIT ( ) );
#3390=ORIENTED_EDGE ( 'NONE', *, *, #1185, .T. ) ;
#3393=DIRECTION ( 'NONE',  ( -1.000000000000000000, -0.000000000000000000, -0.000000000000000000 ) ) ;
#3400=CARTESIAN_POINT ( 'NONE',  ( 55.00000000000000711, 75.00000000000000000, 27.50000000000000000 ) ) ;
#3405=VECTOR ( 'NONE', #4363, 1000.000000000000000 ) ;
#3424=CARTESIAN_POINT ( 'NONE',  ( -75.00000000000000000, -75.00000000000000000, -27.50000000000000000 ) ) ;
#3429=ORIENTED_EDGE ( 'NONE', *, *, #3873, .T. ) ;
#3436=DIRECTION ( 'NONE',  ( 1.000000000000000000, 0.000000000000000000, 0.000000000000000000 ) ) ;
#3442=MANIFOLD_SOLID_BREP ( 'Chamfer1', #5981 ) ;
#3446=CARTESIAN_POINT ( 'NONE',  ( -54.99999999999999289, -75.00000000000000000, 27.50000000000000000 ) ) ;
#3453=CARTESIAN_POINT ( 'NONE',  ( 49.00000000000000711, 55.00000000000000711, -27.50000000000000000 ) ) ;
#3494=CARTESIAN_POINT ( 'NONE',  ( 55.00000000000000711, 54.99999999999999289, 27.50000000000000000 ) ) ;
#3532=ORIENTED_EDGE ( 'NONE', *, *, #2345, .F. ) ;
#3541=DIRECTION ( 'NONE',  ( 0.000000000000000000, 0.000000000000000000, 1.000000000000000000 ) ) ;
#3553=FACE_OUTER_BOUND ( 'NONE', #7625, .T. ) ;
#3558=CARTESIAN_POINT ( 'NONE',  ( 99.49999999999998579, 0.000000000000000000, 0.000000000000000000 ) ) ;
#3563=CARTESIAN_POINT ( 'NONE',  ( 60.99999999999998579, 55.00000000000000711, 27.50000000000000000 ) ) ;
#3577=ORIENTED_EDGE ( 'NONE', *, *, #5620, .F. ) ;
#3581=EDGE_LOOP ( 'NONE', ( #3633, #301, #5971, #5429 ) ) ;
#3587=( GEOMETRIC_REPRESENTATION_CONTEXT ( 3 ) GLOBAL_UNCERTAINTY_ASSIGNED_CONTEXT ( ( #8182 ) ) GLOBAL_UNIT_ASSIGNED_CONTEXT ( ( #4572, #7156, #2146 ) ) REPRESENTATION_CONTEXT ( 'NONE', 'WORKASPACE' ) );
#3592=VECTOR ( 'NONE', #1405, 1000.000000000000000 ) ;
#3603=DIRECTION ( 'NONE',  ( 1.000000000000000000, 0.000000000000000000, 0.000000000000000000 ) ) ;
#3616=ORIENTED_EDGE ( 'NONE', *, *, #2080, .F. ) ;
#3624=EDGE_LOOP ( 'NONE', ( #8047, #4455, #3673, #914 ) ) ;
#3629=CARTESIAN_POINT ( 'NONE',  ( 99.49999999999998579, 0.000000000000000000, 0.000000000000000000 ) ) ;
#3630=EDGE_LOOP ( 'NONE', ( #6999, #499, #3813, #1609 ) ) ;
#3633=ORIENTED_EDGE ( 'NONE', *, *, #7635, .F. ) ;
#3670=CARTESIAN_POINT ( 'NONE',  ( -75.00000000000000000, -54.99999999999999289, -27.50000000000000000 ) ) ;
#3673=ORIENTED_EDGE ( 'NONE', *, *, #8169, .T. ) ;
#3676=CYLINDRICAL_SURFACE ( 'NONE', #6020, 5.999999999999991118 ) ;
#3696=VERTEX_POINT ( 'NONE', #6637 ) ;
#3700=CARTESIAN_POINT ( 'NONE',  ( 102.5000000000000000, 1.530808498934191521E-15, -12.50000000000000000 ) ) ;
#3715=AXIS2_PLACEMENT_3D ( 'NONE', #2076, #5420, #7238 ) ;
#3731=DIRECTION ( 'NONE',  ( -0.000000000000000000, -0.000000000000000000, 1.000000000000000000 ) ) ;
#3741=AXIS2_PLACEMENT_3D ( 'NONE', #2883, #1635, #8226 ) ;
#3743=ORIENTED_EDGE ( 'NONE', *, *, #5355, .T. ) ;
#3745=VERTEX_POINT ( 'NONE', #3280 ) ;
#3748=CARTESIAN_POINT ( 'NONE',  ( -75.00000000000000000, 75.00000000000000000, -27.50000000000000000 ) ) ;
#3761=EDGE_CURVE ( 'NONE', #3972, #7231, #2817, .T. ) ;
#3777=AXIS2_PLACEMENT_3D ( 'NONE', #2673, #5249, #4006 ) ;
#3782=EDGE_CURVE ( 'NONE', #2265, #2372, #1715, .T. ) ;
#3790=UNCERTAINTY_MEASURE_WITH_UNIT (LENGTH_MEASURE( 1.000000000000000082E-05 ), #6519, 'distance_accuracy_value', 'NONE');
#3792=DIRECTION ( 'NONE',  ( 1.000000000000000000, 0.000000000000000000, 0.000000000000000000 ) ) ;
#3794=DIRECTION ( 'NONE',  ( 0.000000000000000000, -0.000000000000000000, -1.000000000000000000 ) ) ;
#3812=DIRECTION ( 'NONE',  ( 0.000000000000000000, 1.000000000000000000, 0.000000000000000000 ) ) ;
#3813=ORIENTED_EDGE ( 'NONE', *, *, #5462, .T. ) ;
#3815=ORIENTED_EDGE ( 'NONE', *, *, #3761, .T. ) ;
#3820=CARTESIAN_POINT ( 'NONE',  ( -49.00000000000000711, -55.00000000000000711, -27.50000000000000000 ) ) ;
#3822=FACE_OUTER_BOUND ( 'NONE', #3186, .T. ) ;
#3839=CIRCLE ( 'NONE', #4905, 20.00000000000000355 ) ;
#3843=EDGE_LOOP ( 'NONE', ( #596, #1363, #7477, #5706, #5134, #4064, #4973, #6420 ) ) ;
#3873=EDGE_CURVE ( 'NONE', #3094, #66, #4336, .T. ) ;
#3888=FACE_BOUND ( 'NONE', #16, .T. ) ;
#3899=VECTOR ( 'NONE', #532, 1000.000000000000000 ) ;
#3903=CYLINDRICAL_SURFACE ( 'NONE', #4427, 12.50000000000000000 ) ;
#3904=AXIS2_PLACEMENT_3D ( 'NONE', #2269, #7410, #1625 ) ;
#3906=CIRCLE ( 'NONE', #7697, 12.50000000000000000 ) ;
#3928=DIRECTION ( 'NONE',  ( 1.000000000000000000, 0.000000000000000000, 0.000000000000000000 ) ) ;
#3929=DIRECTION ( 'NONE',  ( -0.000000000000000000, -0.000000000000000000, 1.000000000000000000 ) ) ;
#3934=VERTEX_POINT ( 'NONE', #4864 ) ;
#3937=PLANE ( 'NONE',  #1599 ) ;
#3957=CARTESIAN_POINT ( 'NONE',  ( 99.49999999999998579, 0.000000000000000000, 0.000000000000000000 ) ) ;
#3959=CARTESIAN_POINT ( 'NONE',  ( -75.00000000000000000, 0.000000000000000000, 0.000000000000000000 ) ) ;
#3969=CYLINDRICAL_SURFACE ( 'NONE', #4703, 5.999999999999991118 ) ;
#3972=VERTEX_POINT ( 'NONE', #2480 ) ;
#3983=CYLINDRICAL_SURFACE ( 'NONE', #6229, 5.999999999999991118 ) ;
#3996=CARTESIAN_POINT ( 'NONE',  ( 49.00000000000000000, 55.00000000000000711, 27.50000000000000000 ) ) ;
#3997=CARTESIAN_POINT ( 'NONE',  ( 55.00000000000000711, 54.99999999999999289, -27.50000000000000000 ) ) ;
#4006=DIRECTION ( 'NONE',  ( 0.000000000000000000, 0.000000000000000000, 1.000000000000000000 ) ) ;
#4023=EDGE_CURVE ( 'NONE', #7555, #7110, #1177, .T. ) ;
#4038=CARTESIAN_POINT ( 'NONE',  ( 75.00000000000000000, -75.00000000000000000, 27.50000000000000000 ) ) ;
#4040=CYLINDRICAL_SURFACE ( 'NONE', #5636, 20.00000000000000355 ) ;
#4044=DIRECTION ( 'NONE',  ( 0.000000000000000000, 0.000000000000000000, -1.000000000000000000 ) ) ;
#4050=CIRCLE ( 'NONE', #277, 12.50000000000000000 ) ;
#4064=ORIENTED_EDGE ( 'NONE', *, *, #4299, .T. ) ;
#4076=VERTEX_POINT ( 'NONE', #6260 ) ;
#4077=CARTESIAN_POINT ( 'NONE',  ( 102.5000000000000000, 1.530808498934191521E-15, -12.50000000000000000 ) ) ;
#4084=CARTESIAN_POINT ( 'NONE',  ( 75.00000000000000000, 1.530808498934191521E-15, -12.50000000000000000 ) ) ;
#4116=CARTESIAN_POINT ( 'NONE',  ( 55.00000000000000711, 75.00000000000000000, -27.50000000000000000 ) ) ;
#4129=AXIS2_PLACEMENT_3D ( 'NONE', #5629, #2267, #4988 ) ;
#4151=EDGE_CURVE ( 'NONE', #4528, #8051, #5759, .T. ) ;
#4155=AXIS2_PLACEMENT_3D ( 'NONE', #6677, #4765, #2863 ) ;
#4227=ORIENTED_EDGE ( 'NONE', *, *, #6450, .F. ) ;
#4241=DIRECTION ( 'NONE',  ( -0.000000000000000000, -0.000000000000000000, 1.000000000000000000 ) ) ;
#4245=VERTEX_POINT ( 'NONE', #3820 ) ;
#4246=ADVANCED_FACE ( 'NONE', ( #5123 ), #5209, .T. ) ;
#4247=EDGE_CURVE ( 'NONE', #4245, #8175, #86, .T. ) ;
#4250=CARTESIAN_POINT ( 'NONE',  ( -49.00000000000000000, 55.00000000000000711, 27.50000000000000000 ) ) ;
#4256=DIRECTION ( 'NONE',  ( 1.000000000000000000, 0.000000000000000000, 0.000000000000000000 ) ) ;
#4258=DIRECTION ( 'NONE',  ( 1.000000000000000000, 0.000000000000000000, 0.000000000000000000 ) ) ;
#4270=ORIENTED_EDGE ( 'NONE', *, *, #7626, .T. ) ;
#4280=PRODUCT_CONTEXT ( 'NONE', #8297, 'mechanical' ) ;
#4291=LINE ( 'NONE', #1068, #5903 ) ;
#4294=VECTOR ( 'NONE', #2138, 1000.000000000000000 ) ;
#4297=PRODUCT ( 'Probe head motor', 'Probe head motor', '', ( #4280 ) ) ;
#4298=CARTESIAN_POINT ( 'NONE',  ( 75.00000000000000000, -75.00000000000000000, 27.50000000000000000 ) ) ;
#4299=EDGE_CURVE ( 'NONE', #4717, #110, #7112, .T. ) ;
#4311=CYLINDRICAL_SURFACE ( 'NONE', #3324, 20.00000000000000355 ) ;
#4312=ORIENTED_EDGE ( 'NONE', *, *, #5355, .F. ) ;
#4316=DIRECTION ( 'NONE',  ( -1.000000000000000000, -0.000000000000000000, -0.000000000000000000 ) ) ;
#4325=ORIENTED_EDGE ( 'NONE', *, *, #6182, .T. ) ;
#4336=LINE ( 'NONE', #7749, #7800 ) ;
#4337=ORIENTED_EDGE ( 'NONE', *, *, #5620, .T. ) ;
#4341=LINE ( 'NONE', #4298, #6735 ) ;
#4363=DIRECTION ( 'NONE',  ( -1.000000000000000000, -0.000000000000000000, -0.000000000000000000 ) ) ;
#4377=VERTEX_POINT ( 'NONE', #2110 ) ;
#4390=CARTESIAN_POINT ( 'NONE',  ( -54.99999999999999289, -54.99999999999999289, 27.50000000000000000 ) ) ;
#4400=ORIENTED_EDGE ( 'NONE', *, *, #5871, .T. ) ;
#4407=ADVANCED_FACE ( 'NONE', ( #3371 ), #1159, .F. ) ;
#4420=EDGE_CURVE ( 'NONE', #8051, #4528, #2538, .T. ) ;
#4426=CARTESIAN_POINT ( 'NONE',  ( 102.5000000000000000, 0.000000000000000000, 0.000000000000000000 ) ) ;
#4427=AXIS2_PLACEMENT_3D ( 'NONE', #5170, #7763, #1983 ) ;
#4453=DIRECTION ( 'NONE',  ( 1.000000000000000000, 0.000000000000000000, 0.000000000000000000 ) ) ;
#4455=ORIENTED_EDGE ( 'NONE', *, *, #6307, .T. ) ;
#4476=ORIENTED_EDGE ( 'NONE', *, *, #1867, .F. ) ;
#4482=CARTESIAN_POINT ( 'NONE',  ( -49.00000000000000000, -55.00000000000000711, 27.50000000000000000 ) ) ;
#4483=LINE ( 'NONE', #7073, #7893 ) ;
#4497=CARTESIAN_POINT ( 'NONE',  ( 75.00000000000000000, 0.000000000000000000, 0.000000000000000000 ) ) ;
#4501=EDGE_CURVE ( 'NONE', #110, #1626, #1117, .T. ) ;
#4504=DIRECTION ( 'NONE',  ( -0.000000000000000000, -0.000000000000000000, 1.000000000000000000 ) ) ;
#4511=ADVANCED_FACE ( 'NONE', ( #518 ), #3676, .F. ) ;
#4521=DIRECTION ( 'NONE',  ( -0.000000000000000000, -0.000000000000000000, 1.000000000000000000 ) ) ;
#4522=VECTOR ( 'NONE', #6832, 1000.000000000000000 ) ;
#4528=VERTEX_POINT ( 'NONE', #4250 ) ;
#4534=DIRECTION ( 'NONE',  ( 1.000000000000000000, 0.000000000000000000, 0.000000000000000000 ) ) ;
#4550=AXIS2_PLACEMENT_3D ( 'NONE', #4038, #6625, #847 ) ;
#4572=( LENGTH_UNIT ( ) NAMED_UNIT ( * ) SI_UNIT ( .MILLI., .METRE. ) );
#4574=CIRCLE ( 'NONE', #2819, 12.50000000000000000 ) ;
#4605=ORIENTED_EDGE ( 'NONE', *, *, #5514, .T. ) ;
#4624=ORIENTED_EDGE ( 'NONE', *, *, #2348, .T. ) ;
#4655=FACE_OUTER_BOUND ( 'NONE', #1731, .T. ) ;
#4657=CIRCLE ( 'NONE', #2878, 5.999999999999984901 ) ;
#4662=FACE_OUTER_BOUND ( 'NONE', #7403, .T. ) ;
#4669=CARTESIAN_POINT ( 'NONE',  ( -99.49999999999998579, 1.530808498934191521E-15, -12.50000000000000000 ) ) ;
#4678=FACE_BOUND ( 'NONE', #1476, .T. ) ;
#4687=ADVANCED_FACE ( 'NONE', ( #5071 ), #8252, .T. ) ;
#4689=ORIENTED_EDGE ( 'NONE', *, *, #1543, .T. ) ;
#4703=AXIS2_PLACEMENT_3D ( 'NONE', #6548, #7444, #1694 ) ;
#4715=ORIENTED_EDGE ( 'NONE', *, *, #7209, .T. ) ;
#4717=VERTEX_POINT ( 'NONE', #200 ) ;
#4718=DIRECTION ( 'NONE',  ( -0.000000000000000000, -0.000000000000000000, 1.000000000000000000 ) ) ;
#4755=ORIENTED_EDGE ( 'NONE', *, *, #5208, .T. ) ;
#4765=DIRECTION ( 'NONE',  ( -0.000000000000000000, -0.000000000000000000, 1.000000000000000000 ) ) ;
#4773=EDGE_CURVE ( 'NONE', #6358, #7231, #7269, .T. ) ;
#4777=DIRECTION ( 'NONE',  ( -0.000000000000000000, -0.000000000000000000, 1.000000000000000000 ) ) ;
#4780=LINE ( 'NONE', #2722, #1800 ) ;
#4801=DIRECTION ( 'NONE',  ( 1.000000000000000000, -1.734723475976806700E-15, 0.000000000000000000 ) ) ;
#4806=PLANE ( 'NONE',  #5382 ) ;
#4814=DIRECTION ( 'NONE',  ( -0.000000000000000000, -0.000000000000000000, 1.000000000000000000 ) ) ;
#4831=CIRCLE ( 'NONE', #1214, 5.999999999999984901 ) ;
#4835=ADVANCED_FACE ( 'NONE', ( #246 ), #4040, .T. ) ;
#4839=AXIS2_PLACEMENT_3D ( 'NONE', #6073, #2827, #1492 ) ;
#4864=CARTESIAN_POINT ( 'NONE',  ( 99.49999999999998579, 0.000000000000000000, 12.50000000000000000 ) ) ;
#4869=ORIENTED_EDGE ( 'NONE', *, *, #5944, .T. ) ;
#4873=ORIENTED_EDGE ( 'NONE', *, *, #1392, .F. ) ;
#4878=PRODUCT_DEFINITION_CONTEXT ( 'detailed design', #6511, 'design' ) ;
#4894=LINE ( 'NONE', #4928, #6431 ) ;
#4898=ORIENTED_EDGE ( 'NONE', *, *, #5761, .F. ) ;
#4902=EDGE_CURVE ( 'NONE', #4377, #8051, #4894, .T. ) ;
#4904=DIRECTION ( 'NONE',  ( -0.000000000000000000, -0.000000000000000000, 1.000000000000000000 ) ) ;
#4905=AXIS2_PLACEMENT_3D ( 'NONE', #5381, #3541, #1461 ) ;
#4907=CARTESIAN_POINT ( 'NONE',  ( -54.99999999999999289, 55.00000000000000711, 27.50000000000000000 ) ) ;
#4908=ORIENTED_EDGE ( 'NONE', *, *, #2229, .T. ) ;
#4922=EDGE_LOOP ( 'NONE', ( #760, #4715, #4908, #5105 ) ) ;
#4925=( GEOMETRIC_REPRESENTATION_CONTEXT ( 3 ) GLOBAL_UNCERTAINTY_ASSIGNED_CONTEXT ( ( #3790 ) ) GLOBAL_UNIT_ASSIGNED_CONTEXT ( ( #6519, #7919, #3379 ) ) REPRESENTATION_CONTEXT ( 'NONE', 'WORKASPACE' ) );
#4928=CARTESIAN_POINT ( 'NONE',  ( -60.99999999999998579, 55.00000000000000711, 27.50000000000000000 ) ) ;
#4931=ORIENTED_EDGE ( 'NONE', *, *, #8169, .F. ) ;
#4946=AXIS2_PLACEMENT_3D ( 'NONE', #7151, #1377, #6385 ) ;
#4954=VERTEX_POINT ( 'NONE', #420 ) ;
#4973=ORIENTED_EDGE ( 'NONE', *, *, #4501, .T. ) ;
#4988=DIRECTION ( 'NONE',  ( 0.000000000000000000, -0.000000000000000000, 1.000000000000000000 ) ) ;
#5009=ORIENTED_EDGE ( 'NONE', *, *, #7439, .F. ) ;
#5051=ORIENTED_EDGE ( 'NONE', *, *, #512, .F. ) ;
#5067=DIRECTION ( 'NONE',  ( -1.000000000000000000, -0.000000000000000000, -0.000000000000000000 ) ) ;
#5071=FACE_OUTER_BOUND ( 'NONE', #1295, .T. ) ;
#5094=CARTESIAN_POINT ( 'NONE',  ( 60.99999999999998579, -55.00000000000000711, 27.50000000000000000 ) ) ;
#5102=CIRCLE ( 'NONE', #1066, 12.50000000000000000 ) ;
#5105=ORIENTED_EDGE ( 'NONE', *, *, #863, .T. ) ;
#5123=FACE_OUTER_BOUND ( 'NONE', #8185, .T. ) ;
#5133=ORIENTED_EDGE ( 'NONE', *, *, #1542, .T. ) ;
#5134=ORIENTED_EDGE ( 'NONE', *, *, #7716, .T. ) ;
#5136=ORIENTED_EDGE ( 'NONE', *, *, #8326, .F. ) ;
#5149=EDGE_CURVE ( 'NONE', #8000, #6145, #236, .T. ) ;
#5156=DIRECTION ( 'NONE',  ( 1.000000000000000000, 0.000000000000000000, 0.000000000000000000 ) ) ;
#5166=DIRECTION ( 'NONE',  ( 0.000000000000000000, -1.000000000000000000, 0.000000000000000000 ) ) ;
#5170=CARTESIAN_POINT ( 'NONE',  ( 102.5000000000000000, 0.000000000000000000, 0.000000000000000000 ) ) ;
#5185=CARTESIAN_POINT ( 'NONE',  ( -99.49999999999998579, 0.000000000000000000, 0.000000000000000000 ) ) ;
#5196=ADVANCED_FACE ( 'NONE', ( #5945 ), #2799, .T. ) ;
#5199=DIRECTION ( 'NONE',  ( 0.000000000000000000, 0.000000000000000000, 1.000000000000000000 ) ) ;
#5208=EDGE_CURVE ( 'NONE', #8191, #4076, #928, .T. ) ;
#5209=CYLINDRICAL_SURFACE ( 'NONE', #4946, 20.00000000000000355 ) ;
#5211=CARTESIAN_POINT ( 'NONE',  ( 54.99999999999999289, -55.00000000000000711, 27.50000000000000000 ) ) ;
#5218=DIRECTION ( 'NONE',  ( 0.000000000000000000, 0.000000000000000000, -1.000000000000000000 ) ) ;
#5223=DIRECTION ( 'NONE',  ( 0.000000000000000000, 0.000000000000000000, -1.000000000000000000 ) ) ;
#5228=LINE ( 'NONE', #1152, #6433 ) ;
#5240=CARTESIAN_POINT ( 'NONE',  ( -102.5000000000000000, 0.000000000000000000, 0.000000000000000000 ) ) ;
#5243=CARTESIAN_POINT ( 'NONE',  ( -54.99999999999999289, -55.00000000000000711, -27.50000000000000000 ) ) ;
#5249=DIRECTION ( 'NONE',  ( -1.000000000000000000, -0.000000000000000000, -0.000000000000000000 ) ) ;
#5250=ADVANCED_FACE ( 'NONE', ( #1434 ), #7935, .T. ) ;
#5255=FACE_OUTER_BOUND ( 'NONE', #5731, .T. ) ;
#5258=DIRECTION ( 'NONE',  ( 1.000000000000000000, 0.000000000000000000, 0.000000000000000000 ) ) ;
#5286=FACE_BOUND ( 'NONE', #7760, .T. ) ;
#5289=FACE_BOUND ( 'NONE', #2346, .T. ) ;
#5290=CARTESIAN_POINT ( 'NONE',  ( 75.00000000000000000, 0.000000000000000000, 12.50000000000000000 ) ) ;
#5300=DIRECTION ( 'NONE',  ( 0.000000000000000000, 0.000000000000000000, -1.000000000000000000 ) ) ;
#5312=CARTESIAN_POINT ( 'NONE',  ( 60.99999999999998579, 55.00000000000000711, 27.50000000000000000 ) ) ;
#5318=DIRECTION ( 'NONE',  ( 0.000000000000000000, 0.000000000000000000, -1.000000000000000000 ) ) ;
#5328=LINE ( 'NONE', #7911, #4294 ) ;
#5346=EDGE_CURVE ( 'NONE', #7256, #7568, #5644, .T. ) ;
#5355=EDGE_CURVE ( 'NONE', #3934, #5497, #6718, .T. ) ;
#5364=FACE_BOUND ( 'NONE', #2270, .T. ) ;
#5380=SHAPE_REPRESENTATION_RELATIONSHIP ( 'NONE' , 'NONE' ,  #5477, #7858 ) ;
#5381=CARTESIAN_POINT ( 'NONE',  ( -54.99999999999999289, 55.00000000000000711, 27.50000000000000000 ) ) ;
#5382=AXIS2_PLACEMENT_3D ( 'NONE', #3325, #288, #1449 ) ;
#5393=DIRECTION ( 'NONE',  ( -1.000000000000000000, -0.000000000000000000, -0.000000000000000000 ) ) ;
#5414=ORIENTED_EDGE ( 'NONE', *, *, #1980, .F. ) ;
#5417=DIRECTION ( 'NONE',  ( 1.000000000000000000, 0.000000000000000000, 0.000000000000000000 ) ) ;
#5420=DIRECTION ( 'NONE',  ( -1.000000000000000000, 0.000000000000000000, 0.000000000000000000 ) ) ;
#5423=CIRCLE ( 'NONE', #8115, 9.499999999999952038 ) ;
#5424=ORIENTED_EDGE ( 'NONE', *, *, #5208, .F. ) ;
#5429=ORIENTED_EDGE ( 'NONE', *, *, #8001, .F. ) ;
#5432=DIRECTION ( 'NONE',  ( -0.000000000000000000, -0.000000000000000000, 1.000000000000000000 ) ) ;
#5440=PLANE ( 'NONE',  #5786 ) ;
#5444=LINE ( 'NONE', #7348, #3101 ) ;
#5462=EDGE_CURVE ( 'NONE', #7568, #3934, #8315, .T. ) ;
#5470=ORIENTED_EDGE ( 'NONE', *, *, #6534, .F. ) ;
#5477=SHAPE_REPRESENTATION ( 'Probe head motor', ( #1299 ), #4925 ) ;
#5492=MECHANICAL_DESIGN_GEOMETRIC_PRESENTATION_REPRESENTATION('',(#1309),#3587);
#5497=VERTEX_POINT ( 'NONE', #7733 ) ;
#5504=AXIS2_PLACEMENT_3D ( 'NONE', #5899, #2126, #2166 ) ;
#5514=EDGE_CURVE ( 'NONE', #7231, #2252, #6586, .T. ) ;
#5533=VERTEX_POINT ( 'NONE', #5691 ) ;
#5552=CARTESIAN_POINT ( 'NONE',  ( -54.99999999999999289, 75.00000000000000000, 27.50000000000000000 ) ) ;
#5555=FACE_OUTER_BOUND ( 'NONE', #5701, .T. ) ;
#5558=FACE_OUTER_BOUND ( 'NONE', #7124, .T. ) ;
#5560=CIRCLE ( 'NONE', #2337, 20.00000000000000355 ) ;
#5579=DIRECTION ( 'NONE',  ( 0.000000000000000000, 0.000000000000000000, -1.000000000000000000 ) ) ;
#5620=EDGE_CURVE ( 'NONE', #3934, #6145, #7556, .T. ) ;
#5621=LINE ( 'NONE', #2992, #3221 ) ;
#5629=CARTESIAN_POINT ( 'NONE',  ( -75.00000000000000000, -75.00000000000000000, 27.50000000000000000 ) ) ;
#5636=AXIS2_PLACEMENT_3D ( 'NONE', #6629, #7351, #5872 ) ;
#5642=DIRECTION ( 'NONE',  ( 0.000000000000000000, 0.000000000000000000, -1.000000000000000000 ) ) ;
#5644=CIRCLE ( 'NONE', #2028, 9.499999999999952038 ) ;
#5651=VECTOR ( 'NONE', #2202, 1000.000000000000000 ) ;
#5673=EDGE_LOOP ( 'NONE', ( #812, #2235, #4689, #5771 ) ) ;
#5691=CARTESIAN_POINT ( 'NONE',  ( 75.00000000000000000, -54.99999999999999289, 27.50000000000000000 ) ) ;
#5699=VERTEX_POINT ( 'NONE', #7205 ) ;
#5700=DIRECTION ( 'NONE',  ( 0.000000000000000000, 0.000000000000000000, 1.000000000000000000 ) ) ;
#5701=EDGE_LOOP ( 'NONE', ( #1398, #1724 ) ) ;
#5706=ORIENTED_EDGE ( 'NONE', *, *, #1976, .T. ) ;
#5731=EDGE_LOOP ( 'NONE', ( #6572, #1696, #7063, #7470 ) ) ;
#5737=DIRECTION ( 'NONE',  ( -1.000000000000000000, -0.000000000000000000, -0.000000000000000000 ) ) ;
#5750=CIRCLE ( 'NONE', #6556, 20.00000000000000355 ) ;
#5755=ORIENTED_EDGE ( 'NONE', *, *, #7515, .T. ) ;
#5759=CIRCLE ( 'NONE', #2134, 5.999999999999991118 ) ;
#5761=EDGE_CURVE ( 'NONE', #3972, #554, #5102, .T. ) ;
#5766=FACE_OUTER_BOUND ( 'NONE', #3581, .T. ) ;
#5771=ORIENTED_EDGE ( 'NONE', *, *, #8302, .F. ) ;
#5782=AXIS2_PLACEMENT_3D ( 'NONE', #4497, #1149, #5700 ) ;
#5786=AXIS2_PLACEMENT_3D ( 'NONE', #8235, #5166, #3794 ) ;
#5798=VECTOR ( 'NONE', #2911, 1000.000000000000000 ) ;
#5814=ORIENTED_EDGE ( 'NONE', *, *, #2517, .T. ) ;
#5853=ORIENTED_EDGE ( 'NONE', *, *, #921, .T. ) ;
#5856=LINE ( 'NONE', #3424, #5651 ) ;
#5864=ORIENTED_EDGE ( 'NONE', *, *, #1976, .F. ) ;
#5869=DIRECTION ( 'NONE',  ( -0.000000000000000000, 0.000000000000000000, 1.000000000000000000 ) ) ;
#5871=EDGE_CURVE ( 'NONE', #4377, #3745, #4831, .T. ) ;
#5872=DIRECTION ( 'NONE',  ( -1.000000000000000000, 0.000000000000000000, 0.000000000000000000 ) ) ;
#5882=DIRECTION ( 'NONE',  ( -0.000000000000000000, -0.000000000000000000, 1.000000000000000000 ) ) ;
#5883=DIRECTION ( 'NONE',  ( 1.000000000000000000, 0.000000000000000000, 0.000000000000000000 ) ) ;
#5884=CARTESIAN_POINT ( 'NONE',  ( 0.000000000000000000, 0.000000000000000000, 0.000000000000000000 ) ) ;
#5888=CARTESIAN_POINT ( 'NONE',  ( 102.5000000000000000, 0.000000000000000000, 0.000000000000000000 ) ) ;
#5889=ADVANCED_FACE ( 'NONE', ( #8084 ), #2315, .F. ) ;
#5899=CARTESIAN_POINT ( 'NONE',  ( 102.5000000000000000, 0.000000000000000000, 0.000000000000000000 ) ) ;
#5903=VECTOR ( 'NONE', #6719, 1000.000000000000000 ) ;
#5904=EDGE_LOOP ( 'NONE', ( #2066, #388, #3100, #2435, #4931, #976, #1654, #340 ) ) ;
#5908=DIRECTION ( 'NONE',  ( -0.000000000000000000, -0.000000000000000000, -1.000000000000000000 ) ) ;
#5927=DIRECTION ( 'NONE',  ( 1.000000000000000000, 0.000000000000000000, 0.000000000000000000 ) ) ;
#5944=EDGE_CURVE ( 'NONE', #7524, #3696, #384, .T. ) ;
#5945=FACE_OUTER_BOUND ( 'NONE', #3630, .T. ) ;
#5951=CARTESIAN_POINT ( 'NONE',  ( 0.000000000000000000, 0.000000000000000000, -27.50000000000000000 ) ) ;
#5954=CARTESIAN_POINT ( 'NONE',  ( 55.00000000000000711, -75.00000000000000000, 27.50000000000000000 ) ) ;
#5971=ORIENTED_EDGE ( 'NONE', *, *, #3277, .F. ) ;
#5981=CLOSED_SHELL ( 'NONE', ( #7486, #3378, #7314, #3074, #3286, #4511, #7914, #7447, #6697, #1829, #4407, #2018, #6170, #1663, #617, #5250, #4687, #1075, #7218, #3295, #4835, #4246, #5889, #6200, #6167, #1498, #1930, #5196 ) ) ;
#5990=FACE_BOUND ( 'NONE', #6198, .T. ) ;
#6004=DIRECTION ( 'NONE',  ( -0.000000000000000000, -0.000000000000000000, 1.000000000000000000 ) ) ;
#6020=AXIS2_PLACEMENT_3D ( 'NONE', #6252, #4814, #6116 ) ;
#6028=CIRCLE ( 'NONE', #3741, 20.00000000000000355 ) ;
#6033=VECTOR ( 'NONE', #6665, 1000.000000000000000 ) ;
#6036=EDGE_CURVE ( 'NONE', #6639, #7887, #1765, .T. ) ;
#6060=EDGE_LOOP ( 'NONE', ( #5414, #7899, #1959, #4325 ) ) ;
#6073=CARTESIAN_POINT ( 'NONE',  ( -54.99999999999999289, -55.00000000000000711, 27.50000000000000000 ) ) ;
#6082=CARTESIAN_POINT ( 'NONE',  ( 54.99999999999999289, 55.00000000000000711, -27.50000000000000000 ) ) ;
#6089=EDGE_LOOP ( 'NONE', ( #275, #3262, #7135, #7505 ) ) ;
#6116=DIRECTION ( 'NONE',  ( 1.000000000000000000, 0.000000000000000000, 0.000000000000000000 ) ) ;
#6145=VERTEX_POINT ( 'NONE', #5290 ) ;
#6147=DIRECTION ( 'NONE',  ( -0.000000000000000000, -0.000000000000000000, 1.000000000000000000 ) ) ;
#6167=ADVANCED_FACE ( 'NONE', ( #7271 ), #773, .F. ) ;
#6170=ADVANCED_FACE ( 'NONE', ( #2223, #5364, #6631, #5990, #7945 ), #4806, .T. ) ;
#6182=EDGE_CURVE ( 'NONE', #2372, #2265, #7831, .T. ) ;
#6198=EDGE_LOOP ( 'NONE', ( #7301, #7890 ) ) ;
#6200=ADVANCED_FACE ( 'NONE', ( #1406 ), #3969, .F. ) ;
#6220=CARTESIAN_POINT ( 'NONE',  ( -75.00000000000000000, 55.00000000000000711, 27.50000000000000000 ) ) ;
#6229=AXIS2_PLACEMENT_3D ( 'NONE', #7924, #2195, #1589 ) ;
#6245=DIRECTION ( 'NONE',  ( 1.000000000000000000, 0.000000000000000000, 0.000000000000000000 ) ) ;
#6252=CARTESIAN_POINT ( 'NONE',  ( -54.99999999999999289, 55.00000000000000711, 27.50000000000000000 ) ) ;
#6260=CARTESIAN_POINT ( 'NONE',  ( 49.00000000000000000, -55.00000000000000711, 27.50000000000000000 ) ) ;
#6270=VECTOR ( 'NONE', #2488, 1000.000000000000000 ) ;
#6307=EDGE_CURVE ( 'NONE', #110, #6452, #5621, .T. ) ;
#6308=DIRECTION ( 'NONE',  ( 1.000000000000000000, 0.000000000000000000, 0.000000000000000000 ) ) ;
#6322=DIRECTION ( 'NONE',  ( 0.000000000000000000, 0.000000000000000000, 1.000000000000000000 ) ) ;
#6330=LINE ( 'NONE', #7823, #1927 ) ;
#6339=VERTEX_POINT ( 'NONE', #2466 ) ;
#6357=LINE ( 'NONE', #2526, #6635 ) ;
#6358=VERTEX_POINT ( 'NONE', #1361 ) ;
#6385=DIRECTION ( 'NONE',  ( -1.000000000000000000, 0.000000000000000000, 0.000000000000000000 ) ) ;
#6388=CARTESIAN_POINT ( 'NONE',  ( -102.5000000000000000, 0.000000000000000000, 0.000000000000000000 ) ) ;
#6405=ORIENTED_EDGE ( 'NONE', *, *, #8001, .T. ) ;
#6409=CARTESIAN_POINT ( 'NONE',  ( 54.99999999999999289, -54.99999999999999289, -27.50000000000000000 ) ) ;
#6420=ORIENTED_EDGE ( 'NONE', *, *, #885, .T. ) ;
#6425=CARTESIAN_POINT ( 'NONE',  ( -54.99999999999999289, -75.00000000000000000, -27.50000000000000000 ) ) ;
#6431=VECTOR ( 'NONE', #4241, 1000.000000000000000 ) ;
#6432=ORIENTED_EDGE ( 'NONE', *, *, #1134, .F. ) ;
#6433=VECTOR ( 'NONE', #6885, 1000.000000000000000 ) ;
#6438=EDGE_LOOP ( 'NONE', ( #4476, #796, #723, #1689 ) ) ;
#6450=EDGE_CURVE ( 'NONE', #554, #3972, #3906, .T. ) ;
#6452=VERTEX_POINT ( 'NONE', #4116 ) ;
#6456=VECTOR ( 'NONE', #437, 1000.000000000000000 ) ;
#6467=CIRCLE ( 'NONE', #2824, 20.00000000000000355 ) ;
#6469=ORIENTED_EDGE ( 'NONE', *, *, #4773, .T. ) ;
#6470=DIRECTION ( 'NONE',  ( -0.000000000000000000, -0.000000000000000000, 1.000000000000000000 ) ) ;
#6476=EDGE_CURVE ( 'NONE', #5497, #3934, #4574, .T. ) ;
#6497=DIRECTION ( 'NONE',  ( 0.000000000000000000, 0.000000000000000000, -1.000000000000000000 ) ) ;
#6511=APPLICATION_CONTEXT ( 'automotive_design' ) ;
#6512=DIRECTION ( 'NONE',  ( 0.000000000000000000, 0.000000000000000000, -1.000000000000000000 ) ) ;
#6519=( LENGTH_UNIT ( ) NAMED_UNIT ( * ) SI_UNIT ( .MILLI., .METRE. ) );
#6534=EDGE_CURVE ( 'NONE', #6339, #3044, #2699, .T. ) ;
#6539=CARTESIAN_POINT ( 'NONE',  ( 99.49999999999998579, 0.000000000000000000, 0.000000000000000000 ) ) ;
#6540=EDGE_CURVE ( 'NONE', #5497, #8000, #1523, .T. ) ;
#6544=FACE_BOUND ( 'NONE', #734, .T. ) ;
#6548=CARTESIAN_POINT ( 'NONE',  ( 54.99999999999999289, 55.00000000000000711, 27.50000000000000000 ) ) ;
#6549=PRODUCT_DEFINITION_SHAPE ( 'NONE', 'NONE',  #1585 ) ;
#6556=AXIS2_PLACEMENT_3D ( 'NONE', #6409, #75, #5156 ) ;
#6572=ORIENTED_EDGE ( 'NONE', *, *, #6902, .T. ) ;
#6582=AXIS2_PLACEMENT_3D ( 'NONE', #2737, #2664, #35 ) ;
#6586=CIRCLE ( 'NONE', #2686, 12.50000000000000000 ) ;
#6596=AXIS2_PLACEMENT_3D ( 'NONE', #4390, #3105, #1216 ) ;
#6608=DIRECTION ( 'NONE',  ( 1.000000000000000000, 0.000000000000000000, 0.000000000000000000 ) ) ;
#6611=DIRECTION ( 'NONE',  ( 1.000000000000000000, 0.000000000000000000, 0.000000000000000000 ) ) ;
#6625=DIRECTION ( 'NONE',  ( -1.000000000000000000, 0.000000000000000000, 0.000000000000000000 ) ) ;
#6627=DIRECTION ( 'NONE',  ( 1.000000000000000000, 0.000000000000000000, 0.000000000000000000 ) ) ;
#6629=CARTESIAN_POINT ( 'NONE',  ( 55.00000000000000711, 54.99999999999999289, 27.50000000000000000 ) ) ;
#6631=FACE_BOUND ( 'NONE', #956, .T. ) ;
#6635=VECTOR ( 'NONE', #582, 1000.000000000000000 ) ;
#6637=CARTESIAN_POINT ( 'NONE',  ( 60.99999999999997868, 55.00000000000000711, -27.50000000000000000 ) ) ;
#6639=VERTEX_POINT ( 'NONE', #453 ) ;
#6665=DIRECTION ( 'NONE',  ( -1.000000000000000000, -0.000000000000000000, -0.000000000000000000 ) ) ;
#6677=CARTESIAN_POINT ( 'NONE',  ( 54.99999999999999289, 55.00000000000000711, 27.50000000000000000 ) ) ;
#6686=ORIENTED_EDGE ( 'NONE', *, *, #8326, .T. ) ;
#6697=ADVANCED_FACE ( 'NONE', ( #1777 ), #5440, .F. ) ;
#6706=ORIENTED_EDGE ( 'NONE', *, *, #6307, .F. ) ;
#6718=CIRCLE ( 'NONE', #1060, 12.50000000000000000 ) ;
#6719=DIRECTION ( 'NONE',  ( -0.000000000000000000, -0.000000000000000000, 1.000000000000000000 ) ) ;
#6734=DIRECTION ( 'NONE',  ( -0.000000000000000000, -0.000000000000000000, 1.000000000000000000 ) ) ;
#6735=VECTOR ( 'NONE', #3812, 1000.000000000000000 ) ;
#6761=ORIENTED_EDGE ( 'NONE', *, *, #6450, .T. ) ;
#6777=DIRECTION ( 'NONE',  ( 0.000000000000000000, 0.000000000000000000, 1.000000000000000000 ) ) ;
#6784=CIRCLE ( 'NONE', #598, 5.999999999999984901 ) ;
#6802=ORIENTED_EDGE ( 'NONE', *, *, #5149, .F. ) ;
#6808=FACE_OUTER_BOUND ( 'NONE', #764, .T. ) ;
#6815=CIRCLE ( 'NONE', #209, 9.500000000000008882 ) ;
#6820=CARTESIAN_POINT ( 'NONE',  ( -54.99999999999999289, -75.00000000000000000, 27.50000000000000000 ) ) ;
#6825=DIRECTION ( 'NONE',  ( -1.000000000000000000, -0.000000000000000000, -0.000000000000000000 ) ) ;
#6832=DIRECTION ( 'NONE',  ( -1.000000000000000000, -0.000000000000000000, -0.000000000000000000 ) ) ;
#6840=VECTOR ( 'NONE', #8209, 1000.000000000000000 ) ;
#6878=VECTOR ( 'NONE', #2635, 1000.000000000000000 ) ;
#6885=DIRECTION ( 'NONE',  ( -0.000000000000000000, -0.000000000000000000, 1.000000000000000000 ) ) ;
#6902=EDGE_CURVE ( 'NONE', #7887, #3072, #5856, .T. ) ;
#6924=ORIENTED_EDGE ( 'NONE', *, *, #7851, .T. ) ;
#6941=AXIS2_PLACEMENT_3D ( 'NONE', #1169, #531, #7153 ) ;
#6947=PLANE ( 'NONE',  #6941 ) ;
#6955=CARTESIAN_POINT ( 'NONE',  ( 99.49999999999998579, 0.000000000000000000, 12.50000000000000000 ) ) ;
#6986=CONICAL_SURFACE ( 'NONE', #2801, 9.500000000000008882, 0.7853981633974466137 ) ;
#6999=ORIENTED_EDGE ( 'NONE', *, *, #7626, .F. ) ;
#7004=ORIENTED_EDGE ( 'NONE', *, *, #2345, .T. ) ;
#7045=EDGE_LOOP ( 'NONE', ( #2384, #101, #1657, #2941 ) ) ;
#7063=ORIENTED_EDGE ( 'NONE', *, *, #2034, .F. ) ;
#7073=CARTESIAN_POINT ( 'NONE',  ( 75.00000000000000000, 55.00000000000000711, 27.50000000000000000 ) ) ;
#7086=ORIENTED_EDGE ( 'NONE', *, *, #2976, .T. ) ;
#7098=DIRECTION ( 'NONE',  ( -1.000000000000000000, -0.000000000000000000, -0.000000000000000000 ) ) ;
#7104=ORIENTED_EDGE ( 'NONE', *, *, #5346, .F. ) ;
#7110=VERTEX_POINT ( 'NONE', #8088 ) ;
#7112=CIRCLE ( 'NONE', #356, 20.00000000000000355 ) ;
#7117=DIRECTION ( 'NONE',  ( 1.000000000000000000, 0.000000000000000000, 0.000000000000000000 ) ) ;
#7124=EDGE_LOOP ( 'NONE', ( #7755, #2463, #7658, #3616 ) ) ;
#7130=CIRCLE ( 'NONE', #6582, 20.00000000000000355 ) ;
#7135=ORIENTED_EDGE ( 'NONE', *, *, #4420, .T. ) ;
#7145=CARTESIAN_POINT ( 'NONE',  ( -54.99999999999999289, 75.00000000000000000, -27.50000000000000000 ) ) ;
#7149=ORIENTED_EDGE ( 'NONE', *, *, #6476, .T. ) ;
#7151=CARTESIAN_POINT ( 'NONE',  ( -54.99999999999999289, 55.00000000000000711, 27.50000000000000000 ) ) ;
#7153=DIRECTION ( 'NONE',  ( 0.000000000000000000, 0.000000000000000000, -1.000000000000000000 ) ) ;
#7156=( NAMED_UNIT ( * ) PLANE_ANGLE_UNIT ( ) SI_UNIT ( $, .RADIAN. ) );
#7169=CYLINDRICAL_SURFACE ( 'NONE', #1460, 5.999999999999991118 ) ;
#7205=CARTESIAN_POINT ( 'NONE',  ( 75.00000000000000000, -54.99999999999999289, -27.50000000000000000 ) ) ;
#7206=VERTEX_POINT ( 'NONE', #6425 ) ;
#7209=EDGE_CURVE ( 'NONE', #5533, #5699, #8265, .T. ) ;
#7214=DIRECTION ( 'NONE',  ( -0.000000000000000000, -0.000000000000000000, 1.000000000000000000 ) ) ;
#7218=ADVANCED_FACE ( 'NONE', ( #5766 ), #3055, .T. ) ;
#7220=DIRECTION ( 'NONE',  ( 1.000000000000000000, 0.000000000000000000, 0.000000000000000000 ) ) ;
#7231=VERTEX_POINT ( 'NONE', #7589 ) ;
#7236=DIRECTION ( 'NONE',  ( -0.000000000000000000, -0.000000000000000000, 1.000000000000000000 ) ) ;
#7238=DIRECTION ( 'NONE',  ( 0.000000000000000000, 0.000000000000000000, 1.000000000000000000 ) ) ;
#7244=AXIS2_PLACEMENT_3D ( 'NONE', #382, #988, #1749 ) ;
#7249=EDGE_LOOP ( 'NONE', ( #5424, #5009 ) ) ;
#7253=CARTESIAN_POINT ( 'NONE',  ( 49.00000000000000000, 55.00000000000000711, 27.50000000000000000 ) ) ;
#7256=VERTEX_POINT ( 'NONE', #3139 ) ;
#7262=FACE_OUTER_BOUND ( 'NONE', #4922, .T. ) ;
#7269=LINE ( 'NONE', #3322, #3592 ) ;
#7271=FACE_OUTER_BOUND ( 'NONE', #6438, .T. ) ;
#7276=VERTEX_POINT ( 'NONE', #828 ) ;
#7278=CARTESIAN_POINT ( 'NONE',  ( -75.00000000000000000, -75.00000000000000000, 27.50000000000000000 ) ) ;
#7285=DIRECTION ( 'NONE',  ( 1.000000000000000000, 0.000000000000000000, 0.000000000000000000 ) ) ;
#7301=ORIENTED_EDGE ( 'NONE', *, *, #4151, .F. ) ;
#7314=ADVANCED_FACE ( 'NONE', ( #4655 ), #1378, .F. ) ;
#7348=CARTESIAN_POINT ( 'NONE',  ( -75.00000000000000000, -75.00000000000000000, 27.50000000000000000 ) ) ;
#7351=DIRECTION ( 'NONE',  ( 0.000000000000000000, 0.000000000000000000, -1.000000000000000000 ) ) ;
#7387=ORIENTED_EDGE ( 'NONE', *, *, #4023, .F. ) ;
#7403=EDGE_LOOP ( 'NONE', ( #2150, #2985, #7086, #4755 ) ) ;
#7410=DIRECTION ( 'NONE',  ( 0.000000000000000000, 0.000000000000000000, 1.000000000000000000 ) ) ;
#7413=AXIS2_PLACEMENT_3D ( 'NONE', #5211, #7236, #6608 ) ;
#7439=EDGE_CURVE ( 'NONE', #4076, #8191, #2818, .T. ) ;
#7444=DIRECTION ( 'NONE',  ( -0.000000000000000000, -0.000000000000000000, 1.000000000000000000 ) ) ;
#7447=ADVANCED_FACE ( 'NONE', ( #7917 ), #3903, .T. ) ;
#7453=CARTESIAN_POINT ( 'NONE',  ( 102.5000000000000000, 0.000000000000000000, 9.499999999999952038 ) ) ;
#7456=CIRCLE ( 'NONE', #7593, 5.999999999999984901 ) ;
#7457=ORIENTED_EDGE ( 'NONE', *, *, #512, .T. ) ;
#7462=CARTESIAN_POINT ( 'NONE',  ( 54.99999999999999289, -54.99999999999999289, 27.50000000000000000 ) ) ;
#7466=CARTESIAN_POINT ( 'NONE',  ( -75.00000000000000000, -54.99999999999999289, 27.50000000000000000 ) ) ;
#7469=DIRECTION ( 'NONE',  ( 0.000000000000000000, 0.000000000000000000, -1.000000000000000000 ) ) ;
#7470=ORIENTED_EDGE ( 'NONE', *, *, #6036, .T. ) ;
#7477=ORIENTED_EDGE ( 'NONE', *, *, #7944, .T. ) ;
#7486=ADVANCED_FACE ( 'NONE', ( #6808 ), #807, .T. ) ;
#7493=DIRECTION ( 'NONE',  ( 0.000000000000000000, 0.000000000000000000, 1.000000000000000000 ) ) ;
#7495=ORIENTED_EDGE ( 'NONE', *, *, #7944, .F. ) ;
#7505=ORIENTED_EDGE ( 'NONE', *, *, #7851, .F. ) ;
#7515=EDGE_CURVE ( 'NONE', #7206, #3094, #1661, .T. ) ;
#7524=VERTEX_POINT ( 'NONE', #3453 ) ;
#7531=VECTOR ( 'NONE', #5432, 1000.000000000000000 ) ;
#7547=CARTESIAN_POINT ( 'NONE',  ( 75.00000000000000000, -54.99999999999999289, 27.50000000000000000 ) ) ;
#7553=VECTOR ( 'NONE', #8029, 999.9999999999998863 ) ;
#7555=VERTEX_POINT ( 'NONE', #8116 ) ;
#7556=LINE ( 'NONE', #1774, #1472 ) ;
#7568=VERTEX_POINT ( 'NONE', #7453 ) ;
#7589=CARTESIAN_POINT ( 'NONE',  ( -99.49999999999998579, 0.000000000000000000, 12.50000000000000000 ) ) ;
#7591=CYLINDRICAL_SURFACE ( 'NONE', #652, 5.999999999999991118 ) ;
#7593=AXIS2_PLACEMENT_3D ( 'NONE', #5243, #3929, #6627 ) ;
#7603=LINE ( 'NONE', #3446, #1222 ) ;
#7625=EDGE_LOOP ( 'NONE', ( #5864, #2558, #6432, #3368 ) ) ;
#7626=EDGE_CURVE ( 'NONE', #7256, #5497, #257, .T. ) ;
#7635=EDGE_CURVE ( 'NONE', #2500, #836, #3348, .T. ) ;
#7653=AXIS2_PLACEMENT_3D ( 'NONE', #6388, #5883, #5300 ) ;
#7657=AXIS2_PLACEMENT_3D ( 'NONE', #2894, #6147, #4453 ) ;
#7658=ORIENTED_EDGE ( 'NONE', *, *, #3782, .T. ) ;
#7697=AXIS2_PLACEMENT_3D ( 'NONE', #3959, #3436, #5318 ) ;
#7716=EDGE_CURVE ( 'NONE', #5533, #4717, #4341, .T. ) ;
#7723=CARTESIAN_POINT ( 'NONE',  ( -54.99999999999999289, -55.00000000000000711, -27.50000000000000000 ) ) ;
#7727=LINE ( 'NONE', #4482, #6270 ) ;
#7733=CARTESIAN_POINT ( 'NONE',  ( 99.49999999999998579, 1.530808498934191521E-15, -12.50000000000000000 ) ) ;
#7748=FACE_OUTER_BOUND ( 'NONE', #1386, .T. ) ;
#7749=CARTESIAN_POINT ( 'NONE',  ( 55.00000000000000711, -75.00000000000000000, 27.50000000000000000 ) ) ;
#7755=ORIENTED_EDGE ( 'NONE', *, *, #5944, .F. ) ;
#7760=EDGE_LOOP ( 'NONE', ( #6686, #4400 ) ) ;
#7763=DIRECTION ( 'NONE',  ( -1.000000000000000000, -0.000000000000000000, -0.000000000000000000 ) ) ;
#7776=CARTESIAN_POINT ( 'NONE',  ( -54.99999999999999289, -55.00000000000000711, 27.50000000000000000 ) ) ;
#7800=VECTOR ( 'NONE', #4504, 1000.000000000000000 ) ;
#7809=VERTEX_POINT ( 'NONE', #7145 ) ;
#7823=CARTESIAN_POINT ( 'NONE',  ( 75.00000000000000000, -75.00000000000000000, -27.50000000000000000 ) ) ;
#7827=DIRECTION ( 'NONE',  ( 0.000000000000000000, 0.000000000000000000, 1.000000000000000000 ) ) ;
#7831=CIRCLE ( 'NONE', #4155, 5.999999999999991118 ) ;
#7832=FACE_OUTER_BOUND ( 'NONE', #7045, .T. ) ;
#7837=DIRECTION ( 'NONE',  ( 1.000000000000000000, 0.000000000000000000, 0.000000000000000000 ) ) ;
#7851=EDGE_CURVE ( 'NONE', #3745, #4528, #2595, .T. ) ;
#7858=ADVANCED_BREP_SHAPE_REPRESENTATION ( '', ( #3442, #1299 ), #4925 ) ;
#7887=VERTEX_POINT ( 'NONE', #1407 ) ;
#7890=ORIENTED_EDGE ( 'NONE', *, *, #4420, .F. ) ;
#7893=VECTOR ( 'NONE', #1292, 1000.000000000000000 ) ;
#7899=ORIENTED_EDGE ( 'NONE', *, *, #921, .F. ) ;
#7910=AXIS2_PLACEMENT_3D ( 'NONE', #1985, #4521, #7117 ) ;
#7911=CARTESIAN_POINT ( 'NONE',  ( -75.00000000000000000, -75.00000000000000000, 27.50000000000000000 ) ) ;
#7914=ADVANCED_FACE ( 'NONE', ( #693 ), #3249, .T. ) ;
#7917=FACE_OUTER_BOUND ( 'NONE', #1341, .T. ) ;
#7919=( NAMED_UNIT ( * ) PLANE_ANGLE_UNIT ( ) SI_UNIT ( $, .RADIAN. ) );
#7924=CARTESIAN_POINT ( 'NONE',  ( 54.99999999999999289, -55.00000000000000711, 27.50000000000000000 ) ) ;
#7935=CYLINDRICAL_SURFACE ( 'NONE', #5504, 12.50000000000000000 ) ;
#7944=EDGE_CURVE ( 'NONE', #836, #66, #5328, .T. ) ;
#7945=FACE_OUTER_BOUND ( 'NONE', #3843, .T. ) ;
#8000=VERTEX_POINT ( 'NONE', #4084 ) ;
#8001=EDGE_CURVE ( 'NONE', #836, #7206, #7603, .T. ) ;
#8029=DIRECTION ( 'NONE',  ( -0.7071067811865420216, 8.659560562355001884E-17, -0.7071067811865531239 ) ) ;
#8044=DIRECTION ( 'NONE',  ( 1.000000000000000000, 0.000000000000000000, 0.000000000000000000 ) ) ;
#8047=ORIENTED_EDGE ( 'NONE', *, *, #4501, .F. ) ;
#8051=VERTEX_POINT ( 'NONE', #2829 ) ;
#8057=DIRECTION ( 'NONE',  ( -0.000000000000000000, -0.000000000000000000, 1.000000000000000000 ) ) ;
#8058=AXIS2_PLACEMENT_3D ( 'NONE', #3957, #2053, #7827 ) ;
#8084=FACE_OUTER_BOUND ( 'NONE', #138, .T. ) ;
#8088=CARTESIAN_POINT ( 'NONE',  ( 60.99999999999997868, -55.00000000000000711, -27.50000000000000000 ) ) ;
#8099=CARTESIAN_POINT ( 'NONE',  ( 102.5000000000000000, 0.000000000000000000, 0.000000000000000000 ) ) ;
#8111=ORIENTED_EDGE ( 'NONE', *, *, #5761, .T. ) ;
#8115=AXIS2_PLACEMENT_3D ( 'NONE', #5888, #58, #5218 ) ;
#8116=CARTESIAN_POINT ( 'NONE',  ( 49.00000000000000711, -55.00000000000000711, -27.50000000000000000 ) ) ;
#8135=EDGE_CURVE ( 'NONE', #7887, #7809, #6467, .T. ) ;
#8169=EDGE_CURVE ( 'NONE', #6452, #7809, #3151, .T. ) ;
#8175=VERTEX_POINT ( 'NONE', #8319 ) ;
#8182=UNCERTAINTY_MEASURE_WITH_UNIT (LENGTH_MEASURE( 1.000000000000000082E-05 ), #4572, 'distance_accuracy_value', 'NONE');
#8185=EDGE_LOOP ( 'NONE', ( #1948, #2465, #585, #641 ) ) ;
#8189=ORIENTED_EDGE ( 'NONE', *, *, #7439, .T. ) ;
#8191=VERTEX_POINT ( 'NONE', #5094 ) ;
#8199=DIRECTION ( 'NONE',  ( -0.000000000000000000, -0.000000000000000000, 1.000000000000000000 ) ) ;
#8209=DIRECTION ( 'NONE',  ( -1.000000000000000000, -0.000000000000000000, -0.000000000000000000 ) ) ;
#8226=DIRECTION ( 'NONE',  ( 1.000000000000000000, 1.040834085586084059E-15, 0.000000000000000000 ) ) ;
#8235=CARTESIAN_POINT ( 'NONE',  ( -75.00000000000000000, 75.00000000000000000, 27.50000000000000000 ) ) ;
#8252=CYLINDRICAL_SURFACE ( 'NONE', #2677, 12.50000000000000000 ) ;
#8265=LINE ( 'NONE', #7547, #3899 ) ;
#8277=PRODUCT_DEFINITION_FORMATION_WITH_SPECIFIED_SOURCE ( 'ANY', '', #4297, .NOT_KNOWN. ) ;
#8279=DIRECTION ( 'NONE',  ( -0.000000000000000000, -0.000000000000000000, -1.000000000000000000 ) ) ;
#8297=APPLICATION_CONTEXT ( 'automotive_design' ) ;
#8300=CARTESIAN_POINT ( 'NONE',  ( -54.99999999999999289, 55.00000000000000711, 27.50000000000000000 ) ) ;
#8302=EDGE_CURVE ( 'NONE', #4245, #6339, #7727, .T. ) ;
#8315=LINE ( 'NONE', #6955, #2808 ) ;
#8319=CARTESIAN_POINT ( 'NONE',  ( -60.99999999999997868, -55.00000000000000711, -27.50000000000000000 ) ) ;
#8326=EDGE_CURVE ( 'NONE', #3745, #4377, #3171, .T. ) ;
#8380=COLOUR_RGB('Light Blue',0.38,0.62,0.78);
#8381=FILL_AREA_STYLE_COLOUR('',#8380);
#8382=FILL_AREA_STYLE('',(#8381));
#8383=SURFACE_STYLE_FILL_AREA(#8382);
#8384=SURFACE_SIDE_STYLE('',(#8383));
#8385=SURFACE_STYLE_USAGE(.BOTH.,#8384);
#8386=PRESENTATION_STYLE_ASSIGNMENT((#8385));
ENDSEC;
END-ISO-10303-21;
